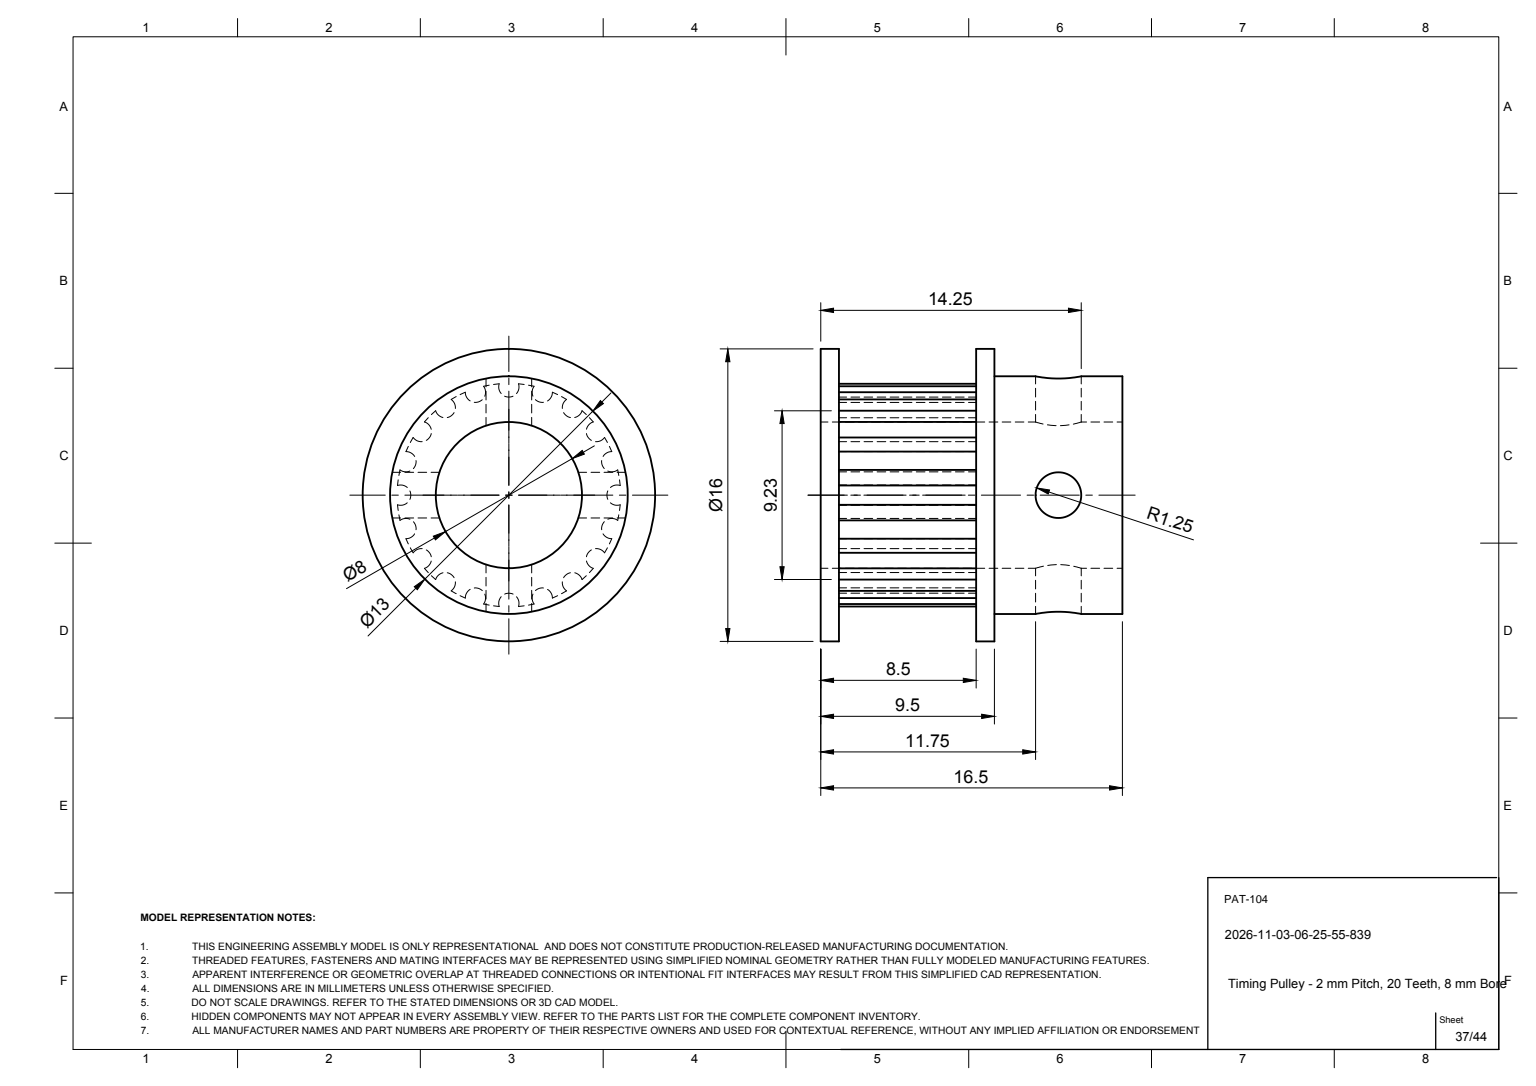
ISO-10303-21;
HEADER;
/* Generated by software containing ST-Developer
 * from STEP Tools, Inc. (www.steptools.com) 
 */

FILE_DESCRIPTION(
/* description */ ('Timing belt drive module 2 mm Pitch Timing 20T-40T'),

/* implementation_level */ '2;1');

FILE_NAME(
/* name */ 'Timing Pulley - 2 mm Pitch, 20 Teeth, 8 mm Bore.step',
/* time_stamp */ '2026-10-28T03:25:12-07:00',
/* author */ (''),
/* organization */ (''),
/* preprocessor_version */ 'ST-DEVELOPER v20.2',
/* originating_system */ 'Autodesk Translation Framework v15.17.0.0',
/* authorisation */ '');

FILE_SCHEMA (('AUTOMOTIVE_DESIGN { 1 0 10303 214 3 1 1 }'));
ENDSEC;

DATA;
#10=MECHANICAL_DESIGN_GEOMETRIC_PRESENTATION_REPRESENTATION('',(#573),#17830);
#341=B_SPLINE_CURVE_WITH_KNOTS('',3,(#16064,#16065,#16066,#16067,#16068,
#16069,#16070,#16071,#16072,#16073),.UNSPECIFIED.,.F.,.F.,(4,2,2,2,4),(0.566550474129931,
0.613761886174531,0.66097329821913,0.708186965196186,0.755400632173242),
 .UNSPECIFIED.);
#342=B_SPLINE_CURVE_WITH_KNOTS('',3,(#16075,#16076,#16077,#16078,#16079,
#16080,#16081,#16082,#16083,#16084,#16085,#16086,#16087,#16088,#16089,#16090,
#16091,#16092),.UNSPECIFIED.,.F.,.F.,(4,2,2,2,2,2,2,2,4),(0.18885015804331,
0.23606157008791,0.283272982132509,0.330486649109565,0.377700316086621,
0.424913983063677,0.472127650040732,0.519339062085332,0.566550474129931),
 .UNSPECIFIED.);
#343=B_SPLINE_CURVE_WITH_KNOTS('',3,(#16093,#16094,#16095,#16096,#16097,
#16098,#16099,#16100,#16101,#16102),.UNSPECIFIED.,.F.,.F.,(4,2,2,2,4),(0.755400632173242,
0.802614299150298,0.849827966127353,0.897039378171953,0.944250790216552),
 .UNSPECIFIED.);
#344=B_SPLINE_CURVE_WITH_KNOTS('',3,(#16106,#16107,#16108,#16109,#16110,
#16111,#16112,#16113,#16114,#16115),.UNSPECIFIED.,.F.,.F.,(4,2,2,2,4),(0.189723673274825,
0.237146208024627,0.28456874277443,0.33200804466204,0.37944734654965),
 .UNSPECIFIED.);
#345=B_SPLINE_CURVE_WITH_KNOTS('',3,(#16117,#16118,#16119,#16120,#16121,
#16122,#16123,#16124,#16125,#16126),.UNSPECIFIED.,.F.,.F.,(4,2,2,2,4),(0.,
0.0474393018876097,0.0948786037752193,0.142301138525022,0.189723673274825),
 .UNSPECIFIED.);
#346=B_SPLINE_CURVE_WITH_KNOTS('',3,(#16128,#16129,#16130,#16131,#16132,
#16133,#16134,#16135,#16136,#16137),.UNSPECIFIED.,.F.,.F.,(4,2,2,2,4),(0.569171019824474,
0.616593554574277,0.66401608932408,0.711455391211689,0.758894693099299),
 .UNSPECIFIED.);
#347=B_SPLINE_CURVE_WITH_KNOTS('',3,(#16138,#16139,#16140,#16141,#16142,
#16143,#16144,#16145,#16146,#16147),.UNSPECIFIED.,.F.,.F.,(4,2,2,2,4),(0.37944734654965,
0.426886648437259,0.474325950324869,0.521748485074671,0.569171019824474),
 .UNSPECIFIED.);
#348=B_SPLINE_CURVE_WITH_KNOTS('',3,(#16151,#16152,#16153,#16154,#16155,
#16156,#16157,#16158,#16159,#16160,#16161,#16162,#16163,#16164,#16165,#16166,
#16167,#16168),.UNSPECIFIED.,.F.,.F.,(4,2,2,2,2,2,2,2,4),(0.,0.0474393018876097,
0.0948786037752194,0.142301138525022,0.189723673274825,0.237146208024628,
0.28456874277443,0.33200804466204,0.37944734654965),.UNSPECIFIED.);
#349=B_SPLINE_CURVE_WITH_KNOTS('',3,(#16169,#16170,#16171,#16172,#16173,
#16174,#16175,#16176,#16177,#16178,#16179,#16180,#16181,#16182,#16183,#16184,
#16185,#16186),.UNSPECIFIED.,.F.,.F.,(4,2,2,2,2,2,2,2,4),(0.37944734654965,
0.426886648437259,0.474325950324869,0.521748485074672,0.569171019824474,
0.616593554574277,0.66401608932408,0.711455391211689,0.758894693099299),
 .UNSPECIFIED.);
#350=B_SPLINE_CURVE_WITH_KNOTS('',3,(#16190,#16191,#16192,#16193,#16194,
#16195,#16196,#16197,#16198,#16199),.UNSPECIFIED.,.F.,.F.,(4,2,2,2,4),(0.566550474129931,
0.613761886174531,0.66097329821913,0.708186965196186,0.755400632173242),
 .UNSPECIFIED.);
#351=B_SPLINE_CURVE_WITH_KNOTS('',3,(#16201,#16202,#16203,#16204,#16205,
#16206,#16207,#16208,#16209,#16210,#16211,#16212,#16213,#16214,#16215,#16216,
#16217,#16218),.UNSPECIFIED.,.F.,.F.,(4,2,2,2,2,2,2,2,4),(0.188850158043311,
0.23606157008791,0.283272982132509,0.330486649109565,0.377700316086621,
0.424913983063677,0.472127650040733,0.519339062085332,0.566550474129931),
 .UNSPECIFIED.);
#352=B_SPLINE_CURVE_WITH_KNOTS('',3,(#16219,#16220,#16221,#16222,#16223,
#16224,#16225,#16226,#16227,#16228),.UNSPECIFIED.,.F.,.F.,(4,2,2,2,4),(0.755400632173242,
0.802614299150298,0.849827966127354,0.897039378171953,0.944250790216552),
 .UNSPECIFIED.);
#353=B_SPLINE_CURVE_WITH_KNOTS('',3,(#16238,#16239,#16240,#16241,#16242,
#16243,#16244,#16245,#16246,#16247,#16248,#16249,#16250,#16251,#16252,#16253,
#16254,#16255),.UNSPECIFIED.,.F.,.F.,(4,2,2,2,2,2,2,2,4),(0.18885015804331,
0.23606157008791,0.283272982132509,0.330486649109565,0.377700316086621,
0.424913983063677,0.472127650040732,0.519339062085332,0.566550474129931),
 .UNSPECIFIED.);
#354=B_SPLINE_CURVE_WITH_KNOTS('',3,(#16257,#16258,#16259,#16260,#16261,
#16262,#16263,#16264,#16265,#16266),.UNSPECIFIED.,.F.,.F.,(4,2,2,2,4),(0.566550474129931,
0.613761886174531,0.66097329821913,0.708186965196186,0.755400632173242),
 .UNSPECIFIED.);
#355=B_SPLINE_CURVE_WITH_KNOTS('',3,(#16267,#16268,#16269,#16270,#16271,
#16272,#16273,#16274,#16275,#16276),.UNSPECIFIED.,.F.,.F.,(4,2,2,2,4),(0.755400632173242,
0.802614299150298,0.849827966127353,0.897039378171953,0.944250790216552),
 .UNSPECIFIED.);
#356=B_SPLINE_CURVE_WITH_KNOTS('',3,(#16279,#16280,#16281,#16282,#16283,
#16284,#16285,#16286,#16287,#16288,#16289,#16290,#16291,#16292,#16293,#16294,
#16295,#16296),.UNSPECIFIED.,.F.,.F.,(4,2,2,2,2,2,2,2,4),(0.188850158043311,
0.23606157008791,0.283272982132509,0.330486649109565,0.377700316086621,
0.424913983063677,0.472127650040733,0.519339062085332,0.566550474129932),
 .UNSPECIFIED.);
#357=B_SPLINE_CURVE_WITH_KNOTS('',3,(#16298,#16299,#16300,#16301,#16302,
#16303,#16304,#16305,#16306,#16307),.UNSPECIFIED.,.F.,.F.,(4,2,2,2,4),(0.566550474129932,
0.613761886174531,0.66097329821913,0.708186965196186,0.755400632173242),
 .UNSPECIFIED.);
#358=B_SPLINE_CURVE_WITH_KNOTS('',3,(#16308,#16309,#16310,#16311,#16312,
#16313,#16314,#16315,#16316,#16317),.UNSPECIFIED.,.F.,.F.,(4,2,2,2,4),(0.755400632173242,
0.802614299150298,0.849827966127354,0.897039378171953,0.944250790216552),
 .UNSPECIFIED.);
#359=B_SPLINE_CURVE_WITH_KNOTS('',3,(#16322,#16323,#16324,#16325,#16326,
#16327,#16328,#16329,#16330,#16331,#16332,#16333,#16334,#16335,#16336,#16337,
#16338,#16339),.UNSPECIFIED.,.F.,.F.,(4,2,2,2,2,2,2,2,4),(0.,0.0474393018876097,
0.0948786037752193,0.142301138525022,0.189723673274825,0.237146208024627,
0.28456874277443,0.33200804466204,0.37944734654965),.UNSPECIFIED.);
#360=B_SPLINE_CURVE_WITH_KNOTS('',3,(#16340,#16341,#16342,#16343,#16344,
#16345,#16346,#16347,#16348,#16349,#16350,#16351,#16352,#16353,#16354,#16355,
#16356,#16357),.UNSPECIFIED.,.F.,.F.,(4,2,2,2,2,2,2,2,4),(0.37944734654965,
0.426886648437259,0.474325950324869,0.521748485074672,0.569171019824474,
0.616593554574277,0.66401608932408,0.711455391211689,0.758894693099299),
 .UNSPECIFIED.);
#361=B_SPLINE_CURVE_WITH_KNOTS('',3,(#16361,#16362,#16363,#16364,#16365,
#16366,#16367,#16368,#16369,#16370,#16371,#16372,#16373,#16374,#16375,#16376,
#16377,#16378),.UNSPECIFIED.,.F.,.F.,(4,2,2,2,2,2,2,2,4),(0.,0.0474393018876097,
0.0948786037752194,0.142301138525022,0.189723673274825,0.237146208024627,
0.28456874277443,0.33200804466204,0.37944734654965),.UNSPECIFIED.);
#362=B_SPLINE_CURVE_WITH_KNOTS('',3,(#16379,#16380,#16381,#16382,#16383,
#16384,#16385,#16386,#16387,#16388,#16389,#16390,#16391,#16392,#16393,#16394,
#16395,#16396),.UNSPECIFIED.,.F.,.F.,(4,2,2,2,2,2,2,2,4),(0.37944734654965,
0.426886648437259,0.474325950324869,0.521748485074672,0.569171019824474,
0.616593554574277,0.66401608932408,0.711455391211689,0.758894693099299),
 .UNSPECIFIED.);
#472=SHAPE_REPRESENTATION_RELATIONSHIP('SRR','None',#18045,#515);
#515=ADVANCED_BREP_SHAPE_REPRESENTATION('',(#629),#17820);
#573=STYLED_ITEM('',(#18331),#629);
#629=MANIFOLD_SOLID_BREP('Body1',#9032);
#741=FACE_BOUND('',#1921,.T.);
#742=FACE_BOUND('',#1922,.T.);
#743=FACE_BOUND('',#1923,.T.);
#744=FACE_BOUND('',#1927,.T.);
#745=FACE_BOUND('',#1928,.T.);
#746=FACE_BOUND('',#1929,.T.);
#747=FACE_BOUND('',#1931,.T.);
#748=FACE_BOUND('',#1933,.T.);
#749=FACE_BOUND('',#1936,.T.);
#750=FACE_BOUND('',#1938,.T.);
#751=FACE_BOUND('',#1941,.T.);
#926=PLANE('',#10269);
#927=PLANE('',#10270);
#928=PLANE('',#10314);
#929=PLANE('',#10315);
#930=PLANE('',#10359);
#1293=FACE_OUTER_BOUND('',#1918,.T.);
#1294=FACE_OUTER_BOUND('',#1919,.T.);
#1295=FACE_OUTER_BOUND('',#1920,.T.);
#1296=FACE_OUTER_BOUND('',#1924,.T.);
#1297=FACE_OUTER_BOUND('',#1925,.T.);
#1298=FACE_OUTER_BOUND('',#1926,.T.);
#1299=FACE_OUTER_BOUND('',#1930,.T.);
#1300=FACE_OUTER_BOUND('',#1932,.T.);
#1301=FACE_OUTER_BOUND('',#1934,.T.);
#1302=FACE_OUTER_BOUND('',#1935,.T.);
#1303=FACE_OUTER_BOUND('',#1937,.T.);
#1304=FACE_OUTER_BOUND('',#1939,.T.);
#1305=FACE_OUTER_BOUND('',#1940,.T.);
#1306=FACE_OUTER_BOUND('',#1942,.T.);
#1307=FACE_OUTER_BOUND('',#1943,.T.);
#1308=FACE_OUTER_BOUND('',#1944,.T.);
#1309=FACE_OUTER_BOUND('',#1945,.T.);
#1310=FACE_OUTER_BOUND('',#1946,.T.);
#1311=FACE_OUTER_BOUND('',#1947,.T.);
#1312=FACE_OUTER_BOUND('',#1948,.T.);
#1313=FACE_OUTER_BOUND('',#1949,.T.);
#1314=FACE_OUTER_BOUND('',#1950,.T.);
#1315=FACE_OUTER_BOUND('',#1951,.T.);
#1316=FACE_OUTER_BOUND('',#1952,.T.);
#1317=FACE_OUTER_BOUND('',#1953,.T.);
#1318=FACE_OUTER_BOUND('',#1954,.T.);
#1319=FACE_OUTER_BOUND('',#1955,.T.);
#1320=FACE_OUTER_BOUND('',#1956,.T.);
#1321=FACE_OUTER_BOUND('',#1957,.T.);
#1322=FACE_OUTER_BOUND('',#1958,.T.);
#1323=FACE_OUTER_BOUND('',#1959,.T.);
#1324=FACE_OUTER_BOUND('',#1960,.T.);
#1325=FACE_OUTER_BOUND('',#1961,.T.);
#1326=FACE_OUTER_BOUND('',#1962,.T.);
#1327=FACE_OUTER_BOUND('',#1963,.T.);
#1328=FACE_OUTER_BOUND('',#1964,.T.);
#1329=FACE_OUTER_BOUND('',#1965,.T.);
#1330=FACE_OUTER_BOUND('',#1966,.T.);
#1331=FACE_OUTER_BOUND('',#1967,.T.);
#1332=FACE_OUTER_BOUND('',#1968,.T.);
#1333=FACE_OUTER_BOUND('',#1969,.T.);
#1334=FACE_OUTER_BOUND('',#1970,.T.);
#1335=FACE_OUTER_BOUND('',#1971,.T.);
#1336=FACE_OUTER_BOUND('',#1972,.T.);
#1337=FACE_OUTER_BOUND('',#1973,.T.);
#1338=FACE_OUTER_BOUND('',#1974,.T.);
#1339=FACE_OUTER_BOUND('',#1975,.T.);
#1340=FACE_OUTER_BOUND('',#1976,.T.);
#1341=FACE_OUTER_BOUND('',#1977,.T.);
#1342=FACE_OUTER_BOUND('',#1978,.T.);
#1343=FACE_OUTER_BOUND('',#1979,.T.);
#1344=FACE_OUTER_BOUND('',#1980,.T.);
#1345=FACE_OUTER_BOUND('',#1981,.T.);
#1918=EDGE_LOOP('',(#7165,#7166,#7167,#7168,#7169,#7170,#7171,#7172,#7173));
#1919=EDGE_LOOP('',(#7174,#7175,#7176,#7177,#7178,#7179,#7180));
#1920=EDGE_LOOP('',(#7181,#7182,#7183,#7184,#7185,#7186,#7187,#7188,#7189));
#1921=EDGE_LOOP('',(#7190,#7191,#7192));
#1922=EDGE_LOOP('',(#7193,#7194,#7195));
#1923=EDGE_LOOP('',(#7196,#7197,#7198));
#1924=EDGE_LOOP('',(#7199,#7200,#7201,#7202,#7203,#7204,#7205));
#1925=EDGE_LOOP('',(#7206,#7207,#7208,#7209,#7210,#7211,#7212));
#1926=EDGE_LOOP('',(#7213,#7214,#7215,#7216,#7217,#7218,#7219,#7220,#7221,
#7222));
#1927=EDGE_LOOP('',(#7223,#7224));
#1928=EDGE_LOOP('',(#7225,#7226));
#1929=EDGE_LOOP('',(#7227,#7228));
#1930=EDGE_LOOP('',(#7229));
#1931=EDGE_LOOP('',(#7230));
#1932=EDGE_LOOP('',(#7231));
#1933=EDGE_LOOP('',(#7232,#7233,#7234,#7235,#7236,#7237,#7238,#7239,#7240,
#7241,#7242,#7243,#7244,#7245,#7246,#7247,#7248,#7249,#7250,#7251,#7252,
#7253,#7254,#7255,#7256,#7257,#7258,#7259,#7260,#7261,#7262,#7263,#7264,
#7265,#7266,#7267,#7268,#7269,#7270,#7271));
#1934=EDGE_LOOP('',(#7272,#7273,#7274,#7275));
#1935=EDGE_LOOP('',(#7276));
#1936=EDGE_LOOP('',(#7277));
#1937=EDGE_LOOP('',(#7278));
#1938=EDGE_LOOP('',(#7279,#7280,#7281,#7282,#7283,#7284,#7285,#7286,#7287,
#7288,#7289,#7290,#7291,#7292,#7293,#7294,#7295,#7296,#7297,#7298,#7299,
#7300,#7301,#7302,#7303,#7304,#7305,#7306,#7307,#7308,#7309,#7310,#7311,
#7312,#7313,#7314,#7315,#7316,#7317,#7318));
#1939=EDGE_LOOP('',(#7319,#7320,#7321,#7322));
#1940=EDGE_LOOP('',(#7323));
#1941=EDGE_LOOP('',(#7324));
#1942=EDGE_LOOP('',(#7325,#7326,#7327,#7328));
#1943=EDGE_LOOP('',(#7329,#7330,#7331,#7332));
#1944=EDGE_LOOP('',(#7333,#7334,#7335,#7336));
#1945=EDGE_LOOP('',(#7337,#7338,#7339,#7340));
#1946=EDGE_LOOP('',(#7341,#7342,#7343,#7344));
#1947=EDGE_LOOP('',(#7345,#7346,#7347,#7348));
#1948=EDGE_LOOP('',(#7349,#7350,#7351,#7352));
#1949=EDGE_LOOP('',(#7353,#7354,#7355,#7356));
#1950=EDGE_LOOP('',(#7357,#7358,#7359,#7360));
#1951=EDGE_LOOP('',(#7361,#7362,#7363,#7364));
#1952=EDGE_LOOP('',(#7365,#7366,#7367,#7368));
#1953=EDGE_LOOP('',(#7369,#7370,#7371,#7372));
#1954=EDGE_LOOP('',(#7373,#7374,#7375,#7376));
#1955=EDGE_LOOP('',(#7377,#7378,#7379,#7380));
#1956=EDGE_LOOP('',(#7381,#7382,#7383,#7384));
#1957=EDGE_LOOP('',(#7385,#7386,#7387,#7388));
#1958=EDGE_LOOP('',(#7389,#7390,#7391,#7392));
#1959=EDGE_LOOP('',(#7393,#7394,#7395,#7396));
#1960=EDGE_LOOP('',(#7397,#7398,#7399,#7400));
#1961=EDGE_LOOP('',(#7401,#7402,#7403,#7404));
#1962=EDGE_LOOP('',(#7405,#7406,#7407,#7408));
#1963=EDGE_LOOP('',(#7409,#7410,#7411,#7412));
#1964=EDGE_LOOP('',(#7413,#7414,#7415,#7416));
#1965=EDGE_LOOP('',(#7417,#7418,#7419,#7420));
#1966=EDGE_LOOP('',(#7421,#7422,#7423,#7424));
#1967=EDGE_LOOP('',(#7425,#7426,#7427,#7428));
#1968=EDGE_LOOP('',(#7429,#7430,#7431,#7432));
#1969=EDGE_LOOP('',(#7433,#7434,#7435,#7436));
#1970=EDGE_LOOP('',(#7437,#7438,#7439,#7440));
#1971=EDGE_LOOP('',(#7441,#7442,#7443,#7444));
#1972=EDGE_LOOP('',(#7445,#7446,#7447,#7448));
#1973=EDGE_LOOP('',(#7449,#7450,#7451,#7452));
#1974=EDGE_LOOP('',(#7453,#7454,#7455,#7456));
#1975=EDGE_LOOP('',(#7457,#7458,#7459,#7460));
#1976=EDGE_LOOP('',(#7461,#7462,#7463,#7464));
#1977=EDGE_LOOP('',(#7465,#7466,#7467,#7468));
#1978=EDGE_LOOP('',(#7469,#7470,#7471,#7472));
#1979=EDGE_LOOP('',(#7473,#7474,#7475,#7476));
#1980=EDGE_LOOP('',(#7477,#7478,#7479,#7480));
#1981=EDGE_LOOP('',(#7481,#7482,#7483,#7484));
#2502=CIRCLE('',#10262,0.65);
#2503=CIRCLE('',#10263,0.65);
#2504=CIRCLE('',#10267,0.4);
#2505=CIRCLE('',#10268,0.4);
#2506=CIRCLE('',#10271,0.8);
#2507=CIRCLE('',#10272,0.0555);
#2508=CIRCLE('',#10273,0.611219772367581);
#2509=CIRCLE('',#10274,0.0555);
#2510=CIRCLE('',#10275,0.611219772367581);
#2511=CIRCLE('',#10276,0.0555);
#2512=CIRCLE('',#10277,0.611219772367581);
#2513=CIRCLE('',#10278,0.0555);
#2514=CIRCLE('',#10279,0.611219772367581);
#2515=CIRCLE('',#10280,0.0555);
#2516=CIRCLE('',#10281,0.611219772367581);
#2517=CIRCLE('',#10282,0.0555);
#2518=CIRCLE('',#10283,0.611219772367581);
#2519=CIRCLE('',#10284,0.0555);
#2520=CIRCLE('',#10285,0.611219772367581);
#2521=CIRCLE('',#10286,0.0555);
#2522=CIRCLE('',#10287,0.611219772367581);
#2523=CIRCLE('',#10288,0.0555);
#2524=CIRCLE('',#10289,0.611219772367581);
#2525=CIRCLE('',#10290,0.0555);
#2526=CIRCLE('',#10291,0.611219772367581);
#2527=CIRCLE('',#10292,0.0555);
#2528=CIRCLE('',#10293,0.611219772367581);
#2529=CIRCLE('',#10294,0.0555);
#2530=CIRCLE('',#10295,0.611219772367581);
#2531=CIRCLE('',#10296,0.0555);
#2532=CIRCLE('',#10297,0.611219772367581);
#2533=CIRCLE('',#10298,0.0555);
#2534=CIRCLE('',#10299,0.611219772367581);
#2535=CIRCLE('',#10300,0.0555);
#2536=CIRCLE('',#10301,0.611219772367581);
#2537=CIRCLE('',#10302,0.0555);
#2538=CIRCLE('',#10303,0.611219772367581);
#2539=CIRCLE('',#10304,0.0555);
#2540=CIRCLE('',#10305,0.611219772367581);
#2541=CIRCLE('',#10306,0.0555);
#2542=CIRCLE('',#10307,0.611219772367581);
#2543=CIRCLE('',#10308,0.0555);
#2544=CIRCLE('',#10309,0.611219772367581);
#2545=CIRCLE('',#10310,0.0555);
#2546=CIRCLE('',#10311,0.611219772367581);
#2547=CIRCLE('',#10313,0.8);
#2548=CIRCLE('',#10316,0.8);
#2549=CIRCLE('',#10317,0.0555);
#2550=CIRCLE('',#10318,0.611219772367581);
#2551=CIRCLE('',#10319,0.0555);
#2552=CIRCLE('',#10320,0.611219772367581);
#2553=CIRCLE('',#10321,0.0555);
#2554=CIRCLE('',#10322,0.611219772367581);
#2555=CIRCLE('',#10323,0.0555);
#2556=CIRCLE('',#10324,0.611219772367581);
#2557=CIRCLE('',#10325,0.0555);
#2558=CIRCLE('',#10326,0.611219772367581);
#2559=CIRCLE('',#10327,0.0555);
#2560=CIRCLE('',#10328,0.611219772367581);
#2561=CIRCLE('',#10329,0.0555);
#2562=CIRCLE('',#10330,0.611219772367581);
#2563=CIRCLE('',#10331,0.0555);
#2564=CIRCLE('',#10332,0.611219772367581);
#2565=CIRCLE('',#10333,0.0555);
#2566=CIRCLE('',#10334,0.611219772367581);
#2567=CIRCLE('',#10335,0.0555);
#2568=CIRCLE('',#10336,0.611219772367581);
#2569=CIRCLE('',#10337,0.0555);
#2570=CIRCLE('',#10338,0.611219772367581);
#2571=CIRCLE('',#10339,0.0555);
#2572=CIRCLE('',#10340,0.611219772367581);
#2573=CIRCLE('',#10341,0.0555);
#2574=CIRCLE('',#10342,0.611219772367581);
#2575=CIRCLE('',#10343,0.0555);
#2576=CIRCLE('',#10344,0.611219772367581);
#2577=CIRCLE('',#10345,0.0555);
#2578=CIRCLE('',#10346,0.611219772367581);
#2579=CIRCLE('',#10347,0.0555);
#2580=CIRCLE('',#10348,0.611219772367581);
#2581=CIRCLE('',#10349,0.0555);
#2582=CIRCLE('',#10350,0.611219772367581);
#2583=CIRCLE('',#10351,0.0555);
#2584=CIRCLE('',#10352,0.611219772367581);
#2585=CIRCLE('',#10353,0.0555);
#2586=CIRCLE('',#10354,0.611219772367581);
#2587=CIRCLE('',#10355,0.0555);
#2588=CIRCLE('',#10356,0.611219772367581);
#2589=CIRCLE('',#10358,0.8);
#3092=LINE('',#16104,#3570);
#3093=LINE('',#16188,#3571);
#3094=LINE('',#16232,#3572);
#3095=LINE('',#16234,#3573);
#3096=LINE('',#16320,#3574);
#3097=LINE('',#16397,#3575);
#3098=LINE('',#16401,#3576);
#3099=LINE('',#16403,#3577);
#3100=LINE('',#16492,#3578);
#3101=LINE('',#16580,#3579);
#3102=LINE('',#16583,#3580);
#3103=LINE('',#16584,#3581);
#3104=LINE('',#16586,#3582);
#3105=LINE('',#16588,#3583);
#3106=LINE('',#16590,#3584);
#3107=LINE('',#16592,#3585);
#3108=LINE('',#16594,#3586);
#3109=LINE('',#16596,#3587);
#3110=LINE('',#16598,#3588);
#3111=LINE('',#16600,#3589);
#3112=LINE('',#16602,#3590);
#3113=LINE('',#16604,#3591);
#3114=LINE('',#16606,#3592);
#3115=LINE('',#16608,#3593);
#3116=LINE('',#16610,#3594);
#3117=LINE('',#16612,#3595);
#3118=LINE('',#16614,#3596);
#3119=LINE('',#16616,#3597);
#3120=LINE('',#16618,#3598);
#3121=LINE('',#16620,#3599);
#3122=LINE('',#16622,#3600);
#3123=LINE('',#16624,#3601);
#3124=LINE('',#16626,#3602);
#3125=LINE('',#16628,#3603);
#3126=LINE('',#16630,#3604);
#3127=LINE('',#16632,#3605);
#3128=LINE('',#16634,#3606);
#3129=LINE('',#16636,#3607);
#3130=LINE('',#16638,#3608);
#3131=LINE('',#16640,#3609);
#3132=LINE('',#16642,#3610);
#3133=LINE('',#16644,#3611);
#3134=LINE('',#16646,#3612);
#3135=LINE('',#16648,#3613);
#3136=LINE('',#16650,#3614);
#3137=LINE('',#16652,#3615);
#3138=LINE('',#16654,#3616);
#3139=LINE('',#16656,#3617);
#3140=LINE('',#16658,#3618);
#3141=LINE('',#16660,#3619);
#3570=VECTOR('',#12599,0.125);
#3571=VECTOR('',#12602,0.125);
#3572=VECTOR('',#12607,0.65);
#3573=VECTOR('',#12608,0.65);
#3574=VECTOR('',#12613,0.125);
#3575=VECTOR('',#12616,0.125);
#3576=VECTOR('',#12621,0.4);
#3577=VECTOR('',#12622,0.4);
#3578=VECTOR('',#12715,0.8);
#3579=VECTOR('',#12806,0.8);
#3580=VECTOR('',#12811,1.);
#3581=VECTOR('',#12812,1.);
#3582=VECTOR('',#12815,1.);
#3583=VECTOR('',#12818,1.);
#3584=VECTOR('',#12821,1.);
#3585=VECTOR('',#12824,1.);
#3586=VECTOR('',#12827,1.);
#3587=VECTOR('',#12830,1.);
#3588=VECTOR('',#12833,1.);
#3589=VECTOR('',#12836,1.);
#3590=VECTOR('',#12839,1.);
#3591=VECTOR('',#12842,1.);
#3592=VECTOR('',#12845,1.);
#3593=VECTOR('',#12848,1.);
#3594=VECTOR('',#12851,1.);
#3595=VECTOR('',#12854,1.);
#3596=VECTOR('',#12857,1.);
#3597=VECTOR('',#12860,1.);
#3598=VECTOR('',#12863,1.);
#3599=VECTOR('',#12866,1.);
#3600=VECTOR('',#12869,1.);
#3601=VECTOR('',#12872,1.);
#3602=VECTOR('',#12875,1.);
#3603=VECTOR('',#12878,1.);
#3604=VECTOR('',#12881,1.);
#3605=VECTOR('',#12884,1.);
#3606=VECTOR('',#12887,1.);
#3607=VECTOR('',#12890,1.);
#3608=VECTOR('',#12893,1.);
#3609=VECTOR('',#12896,1.);
#3610=VECTOR('',#12899,1.);
#3611=VECTOR('',#12902,1.);
#3612=VECTOR('',#12905,1.);
#3613=VECTOR('',#12908,1.);
#3614=VECTOR('',#12911,1.);
#3615=VECTOR('',#12914,1.);
#3616=VECTOR('',#12917,1.);
#3617=VECTOR('',#12920,1.);
#3618=VECTOR('',#12923,1.);
#3619=VECTOR('',#12926,1.);
#4225=VERTEX_POINT('',#16062);
#4226=VERTEX_POINT('',#16063);
#4227=VERTEX_POINT('',#16074);
#4228=VERTEX_POINT('',#16103);
#4229=VERTEX_POINT('',#16105);
#4230=VERTEX_POINT('',#16116);
#4231=VERTEX_POINT('',#16127);
#4232=VERTEX_POINT('',#16149);
#4233=VERTEX_POINT('',#16150);
#4234=VERTEX_POINT('',#16187);
#4235=VERTEX_POINT('',#16189);
#4236=VERTEX_POINT('',#16200);
#4237=VERTEX_POINT('',#16230);
#4238=VERTEX_POINT('',#16233);
#4239=VERTEX_POINT('',#16236);
#4240=VERTEX_POINT('',#16237);
#4241=VERTEX_POINT('',#16256);
#4242=VERTEX_POINT('',#16277);
#4243=VERTEX_POINT('',#16278);
#4244=VERTEX_POINT('',#16297);
#4245=VERTEX_POINT('',#16319);
#4246=VERTEX_POINT('',#16321);
#4247=VERTEX_POINT('',#16359);
#4248=VERTEX_POINT('',#16360);
#4249=VERTEX_POINT('',#16399);
#4250=VERTEX_POINT('',#16402);
#4251=VERTEX_POINT('',#16407);
#4252=VERTEX_POINT('',#16409);
#4253=VERTEX_POINT('',#16410);
#4254=VERTEX_POINT('',#16412);
#4255=VERTEX_POINT('',#16414);
#4256=VERTEX_POINT('',#16416);
#4257=VERTEX_POINT('',#16418);
#4258=VERTEX_POINT('',#16420);
#4259=VERTEX_POINT('',#16422);
#4260=VERTEX_POINT('',#16424);
#4261=VERTEX_POINT('',#16426);
#4262=VERTEX_POINT('',#16428);
#4263=VERTEX_POINT('',#16430);
#4264=VERTEX_POINT('',#16432);
#4265=VERTEX_POINT('',#16434);
#4266=VERTEX_POINT('',#16436);
#4267=VERTEX_POINT('',#16438);
#4268=VERTEX_POINT('',#16440);
#4269=VERTEX_POINT('',#16442);
#4270=VERTEX_POINT('',#16444);
#4271=VERTEX_POINT('',#16446);
#4272=VERTEX_POINT('',#16448);
#4273=VERTEX_POINT('',#16450);
#4274=VERTEX_POINT('',#16452);
#4275=VERTEX_POINT('',#16454);
#4276=VERTEX_POINT('',#16456);
#4277=VERTEX_POINT('',#16458);
#4278=VERTEX_POINT('',#16460);
#4279=VERTEX_POINT('',#16462);
#4280=VERTEX_POINT('',#16464);
#4281=VERTEX_POINT('',#16466);
#4282=VERTEX_POINT('',#16468);
#4283=VERTEX_POINT('',#16470);
#4284=VERTEX_POINT('',#16472);
#4285=VERTEX_POINT('',#16474);
#4286=VERTEX_POINT('',#16476);
#4287=VERTEX_POINT('',#16478);
#4288=VERTEX_POINT('',#16480);
#4289=VERTEX_POINT('',#16482);
#4290=VERTEX_POINT('',#16484);
#4291=VERTEX_POINT('',#16486);
#4292=VERTEX_POINT('',#16490);
#4293=VERTEX_POINT('',#16495);
#4294=VERTEX_POINT('',#16497);
#4295=VERTEX_POINT('',#16498);
#4296=VERTEX_POINT('',#16500);
#4297=VERTEX_POINT('',#16502);
#4298=VERTEX_POINT('',#16504);
#4299=VERTEX_POINT('',#16506);
#4300=VERTEX_POINT('',#16508);
#4301=VERTEX_POINT('',#16510);
#4302=VERTEX_POINT('',#16512);
#4303=VERTEX_POINT('',#16514);
#4304=VERTEX_POINT('',#16516);
#4305=VERTEX_POINT('',#16518);
#4306=VERTEX_POINT('',#16520);
#4307=VERTEX_POINT('',#16522);
#4308=VERTEX_POINT('',#16524);
#4309=VERTEX_POINT('',#16526);
#4310=VERTEX_POINT('',#16528);
#4311=VERTEX_POINT('',#16530);
#4312=VERTEX_POINT('',#16532);
#4313=VERTEX_POINT('',#16534);
#4314=VERTEX_POINT('',#16536);
#4315=VERTEX_POINT('',#16538);
#4316=VERTEX_POINT('',#16540);
#4317=VERTEX_POINT('',#16542);
#4318=VERTEX_POINT('',#16544);
#4319=VERTEX_POINT('',#16546);
#4320=VERTEX_POINT('',#16548);
#4321=VERTEX_POINT('',#16550);
#4322=VERTEX_POINT('',#16552);
#4323=VERTEX_POINT('',#16554);
#4324=VERTEX_POINT('',#16556);
#4325=VERTEX_POINT('',#16558);
#4326=VERTEX_POINT('',#16560);
#4327=VERTEX_POINT('',#16562);
#4328=VERTEX_POINT('',#16564);
#4329=VERTEX_POINT('',#16566);
#4330=VERTEX_POINT('',#16568);
#4331=VERTEX_POINT('',#16570);
#4332=VERTEX_POINT('',#16572);
#4333=VERTEX_POINT('',#16574);
#4334=VERTEX_POINT('',#16578);
#5265=EDGE_CURVE('',#4225,#4226,#341,.T.);
#5266=EDGE_CURVE('',#4227,#4225,#342,.T.);
#5267=EDGE_CURVE('',#4226,#4227,#343,.T.);
#5268=EDGE_CURVE('',#4226,#4228,#3092,.T.);
#5269=EDGE_CURVE('',#4229,#4228,#344,.T.);
#5270=EDGE_CURVE('',#4230,#4229,#345,.T.);
#5271=EDGE_CURVE('',#4231,#4230,#346,.T.);
#5272=EDGE_CURVE('',#4228,#4231,#347,.T.);
#5273=EDGE_CURVE('',#4232,#4233,#348,.T.);
#5274=EDGE_CURVE('',#4233,#4232,#349,.T.);
#5275=EDGE_CURVE('',#4233,#4234,#3093,.T.);
#5276=EDGE_CURVE('',#4235,#4234,#350,.T.);
#5277=EDGE_CURVE('',#4236,#4235,#351,.T.);
#5278=EDGE_CURVE('',#4234,#4236,#352,.T.);
#5279=EDGE_CURVE('',#4237,#4237,#2502,.T.);
#5280=EDGE_CURVE('',#4237,#4227,#3094,.T.);
#5281=EDGE_CURVE('',#4225,#4238,#3095,.T.);
#5282=EDGE_CURVE('',#4238,#4238,#2503,.T.);
#5283=EDGE_CURVE('',#4239,#4240,#353,.T.);
#5284=EDGE_CURVE('',#4240,#4241,#354,.T.);
#5285=EDGE_CURVE('',#4241,#4239,#355,.T.);
#5286=EDGE_CURVE('',#4242,#4243,#356,.T.);
#5287=EDGE_CURVE('',#4243,#4244,#357,.T.);
#5288=EDGE_CURVE('',#4244,#4242,#358,.T.);
#5289=EDGE_CURVE('',#4241,#4245,#3096,.T.);
#5290=EDGE_CURVE('',#4246,#4245,#359,.T.);
#5291=EDGE_CURVE('',#4245,#4246,#360,.T.);
#5292=EDGE_CURVE('',#4247,#4248,#361,.T.);
#5293=EDGE_CURVE('',#4248,#4247,#362,.T.);
#5294=EDGE_CURVE('',#4248,#4244,#3097,.T.);
#5295=EDGE_CURVE('',#4249,#4249,#2504,.T.);
#5296=EDGE_CURVE('',#4249,#4229,#3098,.T.);
#5297=EDGE_CURVE('',#4231,#4250,#3099,.T.);
#5298=EDGE_CURVE('',#4250,#4250,#2505,.T.);
#5299=EDGE_CURVE('',#4251,#4251,#2506,.T.);
#5300=EDGE_CURVE('',#4252,#4253,#2507,.T.);
#5301=EDGE_CURVE('',#4254,#4253,#2508,.T.);
#5302=EDGE_CURVE('',#4254,#4255,#2509,.T.);
#5303=EDGE_CURVE('',#4256,#4255,#2510,.T.);
#5304=EDGE_CURVE('',#4256,#4257,#2511,.T.);
#5305=EDGE_CURVE('',#4258,#4257,#2512,.T.);
#5306=EDGE_CURVE('',#4258,#4259,#2513,.T.);
#5307=EDGE_CURVE('',#4260,#4259,#2514,.T.);
#5308=EDGE_CURVE('',#4260,#4261,#2515,.T.);
#5309=EDGE_CURVE('',#4262,#4261,#2516,.T.);
#5310=EDGE_CURVE('',#4262,#4263,#2517,.T.);
#5311=EDGE_CURVE('',#4264,#4263,#2518,.T.);
#5312=EDGE_CURVE('',#4264,#4265,#2519,.T.);
#5313=EDGE_CURVE('',#4266,#4265,#2520,.T.);
#5314=EDGE_CURVE('',#4266,#4267,#2521,.T.);
#5315=EDGE_CURVE('',#4268,#4267,#2522,.T.);
#5316=EDGE_CURVE('',#4268,#4269,#2523,.T.);
#5317=EDGE_CURVE('',#4270,#4269,#2524,.T.);
#5318=EDGE_CURVE('',#4270,#4271,#2525,.T.);
#5319=EDGE_CURVE('',#4272,#4271,#2526,.T.);
#5320=EDGE_CURVE('',#4272,#4273,#2527,.T.);
#5321=EDGE_CURVE('',#4274,#4273,#2528,.T.);
#5322=EDGE_CURVE('',#4274,#4275,#2529,.T.);
#5323=EDGE_CURVE('',#4276,#4275,#2530,.T.);
#5324=EDGE_CURVE('',#4276,#4277,#2531,.T.);
#5325=EDGE_CURVE('',#4278,#4277,#2532,.T.);
#5326=EDGE_CURVE('',#4278,#4279,#2533,.T.);
#5327=EDGE_CURVE('',#4280,#4279,#2534,.T.);
#5328=EDGE_CURVE('',#4280,#4281,#2535,.T.);
#5329=EDGE_CURVE('',#4282,#4281,#2536,.T.);
#5330=EDGE_CURVE('',#4282,#4283,#2537,.T.);
#5331=EDGE_CURVE('',#4284,#4283,#2538,.T.);
#5332=EDGE_CURVE('',#4284,#4285,#2539,.T.);
#5333=EDGE_CURVE('',#4286,#4285,#2540,.T.);
#5334=EDGE_CURVE('',#4286,#4287,#2541,.T.);
#5335=EDGE_CURVE('',#4288,#4287,#2542,.T.);
#5336=EDGE_CURVE('',#4288,#4289,#2543,.T.);
#5337=EDGE_CURVE('',#4290,#4289,#2544,.T.);
#5338=EDGE_CURVE('',#4290,#4291,#2545,.T.);
#5339=EDGE_CURVE('',#4252,#4291,#2546,.T.);
#5340=EDGE_CURVE('',#4292,#4292,#2547,.T.);
#5341=EDGE_CURVE('',#4292,#4251,#3100,.T.);
#5342=EDGE_CURVE('',#4293,#4293,#2548,.T.);
#5343=EDGE_CURVE('',#4294,#4295,#2549,.T.);
#5344=EDGE_CURVE('',#4295,#4296,#2550,.T.);
#5345=EDGE_CURVE('',#4296,#4297,#2551,.T.);
#5346=EDGE_CURVE('',#4297,#4298,#2552,.T.);
#5347=EDGE_CURVE('',#4298,#4299,#2553,.T.);
#5348=EDGE_CURVE('',#4299,#4300,#2554,.T.);
#5349=EDGE_CURVE('',#4300,#4301,#2555,.T.);
#5350=EDGE_CURVE('',#4301,#4302,#2556,.T.);
#5351=EDGE_CURVE('',#4302,#4303,#2557,.T.);
#5352=EDGE_CURVE('',#4303,#4304,#2558,.T.);
#5353=EDGE_CURVE('',#4304,#4305,#2559,.T.);
#5354=EDGE_CURVE('',#4305,#4306,#2560,.T.);
#5355=EDGE_CURVE('',#4306,#4307,#2561,.T.);
#5356=EDGE_CURVE('',#4307,#4308,#2562,.T.);
#5357=EDGE_CURVE('',#4308,#4309,#2563,.T.);
#5358=EDGE_CURVE('',#4309,#4310,#2564,.T.);
#5359=EDGE_CURVE('',#4310,#4311,#2565,.T.);
#5360=EDGE_CURVE('',#4311,#4312,#2566,.T.);
#5361=EDGE_CURVE('',#4312,#4313,#2567,.T.);
#5362=EDGE_CURVE('',#4313,#4314,#2568,.T.);
#5363=EDGE_CURVE('',#4314,#4315,#2569,.T.);
#5364=EDGE_CURVE('',#4315,#4316,#2570,.T.);
#5365=EDGE_CURVE('',#4316,#4317,#2571,.T.);
#5366=EDGE_CURVE('',#4317,#4318,#2572,.T.);
#5367=EDGE_CURVE('',#4318,#4319,#2573,.T.);
#5368=EDGE_CURVE('',#4319,#4320,#2574,.T.);
#5369=EDGE_CURVE('',#4320,#4321,#2575,.T.);
#5370=EDGE_CURVE('',#4321,#4322,#2576,.T.);
#5371=EDGE_CURVE('',#4322,#4323,#2577,.T.);
#5372=EDGE_CURVE('',#4323,#4324,#2578,.T.);
#5373=EDGE_CURVE('',#4324,#4325,#2579,.T.);
#5374=EDGE_CURVE('',#4325,#4326,#2580,.T.);
#5375=EDGE_CURVE('',#4326,#4327,#2581,.T.);
#5376=EDGE_CURVE('',#4327,#4328,#2582,.T.);
#5377=EDGE_CURVE('',#4328,#4329,#2583,.T.);
#5378=EDGE_CURVE('',#4329,#4330,#2584,.T.);
#5379=EDGE_CURVE('',#4330,#4331,#2585,.T.);
#5380=EDGE_CURVE('',#4331,#4332,#2586,.T.);
#5381=EDGE_CURVE('',#4332,#4333,#2587,.T.);
#5382=EDGE_CURVE('',#4333,#4294,#2588,.T.);
#5383=EDGE_CURVE('',#4334,#4334,#2589,.T.);
#5384=EDGE_CURVE('',#4334,#4293,#3101,.T.);
#5385=EDGE_CURVE('',#4295,#4252,#3102,.T.);
#5386=EDGE_CURVE('',#4253,#4294,#3103,.T.);
#5387=EDGE_CURVE('',#4333,#4254,#3104,.T.);
#5388=EDGE_CURVE('',#4255,#4332,#3105,.T.);
#5389=EDGE_CURVE('',#4331,#4256,#3106,.T.);
#5390=EDGE_CURVE('',#4257,#4330,#3107,.T.);
#5391=EDGE_CURVE('',#4329,#4258,#3108,.T.);
#5392=EDGE_CURVE('',#4259,#4328,#3109,.T.);
#5393=EDGE_CURVE('',#4327,#4260,#3110,.T.);
#5394=EDGE_CURVE('',#4261,#4326,#3111,.T.);
#5395=EDGE_CURVE('',#4325,#4262,#3112,.T.);
#5396=EDGE_CURVE('',#4263,#4324,#3113,.T.);
#5397=EDGE_CURVE('',#4323,#4264,#3114,.T.);
#5398=EDGE_CURVE('',#4265,#4322,#3115,.T.);
#5399=EDGE_CURVE('',#4321,#4266,#3116,.T.);
#5400=EDGE_CURVE('',#4267,#4320,#3117,.T.);
#5401=EDGE_CURVE('',#4319,#4268,#3118,.T.);
#5402=EDGE_CURVE('',#4269,#4318,#3119,.T.);
#5403=EDGE_CURVE('',#4317,#4270,#3120,.T.);
#5404=EDGE_CURVE('',#4271,#4316,#3121,.T.);
#5405=EDGE_CURVE('',#4315,#4272,#3122,.T.);
#5406=EDGE_CURVE('',#4273,#4314,#3123,.T.);
#5407=EDGE_CURVE('',#4313,#4274,#3124,.T.);
#5408=EDGE_CURVE('',#4275,#4312,#3125,.T.);
#5409=EDGE_CURVE('',#4311,#4276,#3126,.T.);
#5410=EDGE_CURVE('',#4277,#4310,#3127,.T.);
#5411=EDGE_CURVE('',#4309,#4278,#3128,.T.);
#5412=EDGE_CURVE('',#4279,#4308,#3129,.T.);
#5413=EDGE_CURVE('',#4307,#4280,#3130,.T.);
#5414=EDGE_CURVE('',#4281,#4306,#3131,.T.);
#5415=EDGE_CURVE('',#4305,#4282,#3132,.T.);
#5416=EDGE_CURVE('',#4283,#4304,#3133,.T.);
#5417=EDGE_CURVE('',#4303,#4284,#3134,.T.);
#5418=EDGE_CURVE('',#4285,#4302,#3135,.T.);
#5419=EDGE_CURVE('',#4301,#4286,#3136,.T.);
#5420=EDGE_CURVE('',#4287,#4300,#3137,.T.);
#5421=EDGE_CURVE('',#4299,#4288,#3138,.T.);
#5422=EDGE_CURVE('',#4289,#4298,#3139,.T.);
#5423=EDGE_CURVE('',#4291,#4296,#3140,.T.);
#5424=EDGE_CURVE('',#4297,#4290,#3141,.T.);
#7165=ORIENTED_EDGE('',*,*,#5265,.F.);
#7166=ORIENTED_EDGE('',*,*,#5266,.F.);
#7167=ORIENTED_EDGE('',*,*,#5267,.F.);
#7168=ORIENTED_EDGE('',*,*,#5268,.T.);
#7169=ORIENTED_EDGE('',*,*,#5269,.F.);
#7170=ORIENTED_EDGE('',*,*,#5270,.F.);
#7171=ORIENTED_EDGE('',*,*,#5271,.F.);
#7172=ORIENTED_EDGE('',*,*,#5272,.F.);
#7173=ORIENTED_EDGE('',*,*,#5268,.F.);
#7174=ORIENTED_EDGE('',*,*,#5273,.F.);
#7175=ORIENTED_EDGE('',*,*,#5274,.F.);
#7176=ORIENTED_EDGE('',*,*,#5275,.T.);
#7177=ORIENTED_EDGE('',*,*,#5276,.F.);
#7178=ORIENTED_EDGE('',*,*,#5277,.F.);
#7179=ORIENTED_EDGE('',*,*,#5278,.F.);
#7180=ORIENTED_EDGE('',*,*,#5275,.F.);
#7181=ORIENTED_EDGE('',*,*,#5279,.F.);
#7182=ORIENTED_EDGE('',*,*,#5280,.T.);
#7183=ORIENTED_EDGE('',*,*,#5266,.T.);
#7184=ORIENTED_EDGE('',*,*,#5281,.T.);
#7185=ORIENTED_EDGE('',*,*,#5282,.F.);
#7186=ORIENTED_EDGE('',*,*,#5281,.F.);
#7187=ORIENTED_EDGE('',*,*,#5265,.T.);
#7188=ORIENTED_EDGE('',*,*,#5267,.T.);
#7189=ORIENTED_EDGE('',*,*,#5280,.F.);
#7190=ORIENTED_EDGE('',*,*,#5277,.T.);
#7191=ORIENTED_EDGE('',*,*,#5276,.T.);
#7192=ORIENTED_EDGE('',*,*,#5278,.T.);
#7193=ORIENTED_EDGE('',*,*,#5283,.T.);
#7194=ORIENTED_EDGE('',*,*,#5284,.T.);
#7195=ORIENTED_EDGE('',*,*,#5285,.T.);
#7196=ORIENTED_EDGE('',*,*,#5286,.T.);
#7197=ORIENTED_EDGE('',*,*,#5287,.T.);
#7198=ORIENTED_EDGE('',*,*,#5288,.T.);
#7199=ORIENTED_EDGE('',*,*,#5284,.F.);
#7200=ORIENTED_EDGE('',*,*,#5283,.F.);
#7201=ORIENTED_EDGE('',*,*,#5285,.F.);
#7202=ORIENTED_EDGE('',*,*,#5289,.T.);
#7203=ORIENTED_EDGE('',*,*,#5290,.F.);
#7204=ORIENTED_EDGE('',*,*,#5291,.F.);
#7205=ORIENTED_EDGE('',*,*,#5289,.F.);
#7206=ORIENTED_EDGE('',*,*,#5292,.F.);
#7207=ORIENTED_EDGE('',*,*,#5293,.F.);
#7208=ORIENTED_EDGE('',*,*,#5294,.T.);
#7209=ORIENTED_EDGE('',*,*,#5287,.F.);
#7210=ORIENTED_EDGE('',*,*,#5286,.F.);
#7211=ORIENTED_EDGE('',*,*,#5288,.F.);
#7212=ORIENTED_EDGE('',*,*,#5294,.F.);
#7213=ORIENTED_EDGE('',*,*,#5295,.F.);
#7214=ORIENTED_EDGE('',*,*,#5296,.T.);
#7215=ORIENTED_EDGE('',*,*,#5269,.T.);
#7216=ORIENTED_EDGE('',*,*,#5272,.T.);
#7217=ORIENTED_EDGE('',*,*,#5297,.T.);
#7218=ORIENTED_EDGE('',*,*,#5298,.F.);
#7219=ORIENTED_EDGE('',*,*,#5297,.F.);
#7220=ORIENTED_EDGE('',*,*,#5271,.T.);
#7221=ORIENTED_EDGE('',*,*,#5270,.T.);
#7222=ORIENTED_EDGE('',*,*,#5296,.F.);
#7223=ORIENTED_EDGE('',*,*,#5273,.T.);
#7224=ORIENTED_EDGE('',*,*,#5274,.T.);
#7225=ORIENTED_EDGE('',*,*,#5292,.T.);
#7226=ORIENTED_EDGE('',*,*,#5293,.T.);
#7227=ORIENTED_EDGE('',*,*,#5290,.T.);
#7228=ORIENTED_EDGE('',*,*,#5291,.T.);
#7229=ORIENTED_EDGE('',*,*,#5279,.T.);
#7230=ORIENTED_EDGE('',*,*,#5295,.T.);
#7231=ORIENTED_EDGE('',*,*,#5299,.T.);
#7232=ORIENTED_EDGE('',*,*,#5300,.T.);
#7233=ORIENTED_EDGE('',*,*,#5301,.F.);
#7234=ORIENTED_EDGE('',*,*,#5302,.T.);
#7235=ORIENTED_EDGE('',*,*,#5303,.F.);
#7236=ORIENTED_EDGE('',*,*,#5304,.T.);
#7237=ORIENTED_EDGE('',*,*,#5305,.F.);
#7238=ORIENTED_EDGE('',*,*,#5306,.T.);
#7239=ORIENTED_EDGE('',*,*,#5307,.F.);
#7240=ORIENTED_EDGE('',*,*,#5308,.T.);
#7241=ORIENTED_EDGE('',*,*,#5309,.F.);
#7242=ORIENTED_EDGE('',*,*,#5310,.T.);
#7243=ORIENTED_EDGE('',*,*,#5311,.F.);
#7244=ORIENTED_EDGE('',*,*,#5312,.T.);
#7245=ORIENTED_EDGE('',*,*,#5313,.F.);
#7246=ORIENTED_EDGE('',*,*,#5314,.T.);
#7247=ORIENTED_EDGE('',*,*,#5315,.F.);
#7248=ORIENTED_EDGE('',*,*,#5316,.T.);
#7249=ORIENTED_EDGE('',*,*,#5317,.F.);
#7250=ORIENTED_EDGE('',*,*,#5318,.T.);
#7251=ORIENTED_EDGE('',*,*,#5319,.F.);
#7252=ORIENTED_EDGE('',*,*,#5320,.T.);
#7253=ORIENTED_EDGE('',*,*,#5321,.F.);
#7254=ORIENTED_EDGE('',*,*,#5322,.T.);
#7255=ORIENTED_EDGE('',*,*,#5323,.F.);
#7256=ORIENTED_EDGE('',*,*,#5324,.T.);
#7257=ORIENTED_EDGE('',*,*,#5325,.F.);
#7258=ORIENTED_EDGE('',*,*,#5326,.T.);
#7259=ORIENTED_EDGE('',*,*,#5327,.F.);
#7260=ORIENTED_EDGE('',*,*,#5328,.T.);
#7261=ORIENTED_EDGE('',*,*,#5329,.F.);
#7262=ORIENTED_EDGE('',*,*,#5330,.T.);
#7263=ORIENTED_EDGE('',*,*,#5331,.F.);
#7264=ORIENTED_EDGE('',*,*,#5332,.T.);
#7265=ORIENTED_EDGE('',*,*,#5333,.F.);
#7266=ORIENTED_EDGE('',*,*,#5334,.T.);
#7267=ORIENTED_EDGE('',*,*,#5335,.F.);
#7268=ORIENTED_EDGE('',*,*,#5336,.T.);
#7269=ORIENTED_EDGE('',*,*,#5337,.F.);
#7270=ORIENTED_EDGE('',*,*,#5338,.T.);
#7271=ORIENTED_EDGE('',*,*,#5339,.F.);
#7272=ORIENTED_EDGE('',*,*,#5340,.F.);
#7273=ORIENTED_EDGE('',*,*,#5341,.T.);
#7274=ORIENTED_EDGE('',*,*,#5299,.F.);
#7275=ORIENTED_EDGE('',*,*,#5341,.F.);
#7276=ORIENTED_EDGE('',*,*,#5340,.T.);
#7277=ORIENTED_EDGE('',*,*,#5282,.T.);
#7278=ORIENTED_EDGE('',*,*,#5342,.F.);
#7279=ORIENTED_EDGE('',*,*,#5343,.T.);
#7280=ORIENTED_EDGE('',*,*,#5344,.T.);
#7281=ORIENTED_EDGE('',*,*,#5345,.T.);
#7282=ORIENTED_EDGE('',*,*,#5346,.T.);
#7283=ORIENTED_EDGE('',*,*,#5347,.T.);
#7284=ORIENTED_EDGE('',*,*,#5348,.T.);
#7285=ORIENTED_EDGE('',*,*,#5349,.T.);
#7286=ORIENTED_EDGE('',*,*,#5350,.T.);
#7287=ORIENTED_EDGE('',*,*,#5351,.T.);
#7288=ORIENTED_EDGE('',*,*,#5352,.T.);
#7289=ORIENTED_EDGE('',*,*,#5353,.T.);
#7290=ORIENTED_EDGE('',*,*,#5354,.T.);
#7291=ORIENTED_EDGE('',*,*,#5355,.T.);
#7292=ORIENTED_EDGE('',*,*,#5356,.T.);
#7293=ORIENTED_EDGE('',*,*,#5357,.T.);
#7294=ORIENTED_EDGE('',*,*,#5358,.T.);
#7295=ORIENTED_EDGE('',*,*,#5359,.T.);
#7296=ORIENTED_EDGE('',*,*,#5360,.T.);
#7297=ORIENTED_EDGE('',*,*,#5361,.T.);
#7298=ORIENTED_EDGE('',*,*,#5362,.T.);
#7299=ORIENTED_EDGE('',*,*,#5363,.T.);
#7300=ORIENTED_EDGE('',*,*,#5364,.T.);
#7301=ORIENTED_EDGE('',*,*,#5365,.T.);
#7302=ORIENTED_EDGE('',*,*,#5366,.T.);
#7303=ORIENTED_EDGE('',*,*,#5367,.T.);
#7304=ORIENTED_EDGE('',*,*,#5368,.T.);
#7305=ORIENTED_EDGE('',*,*,#5369,.T.);
#7306=ORIENTED_EDGE('',*,*,#5370,.T.);
#7307=ORIENTED_EDGE('',*,*,#5371,.T.);
#7308=ORIENTED_EDGE('',*,*,#5372,.T.);
#7309=ORIENTED_EDGE('',*,*,#5373,.T.);
#7310=ORIENTED_EDGE('',*,*,#5374,.T.);
#7311=ORIENTED_EDGE('',*,*,#5375,.T.);
#7312=ORIENTED_EDGE('',*,*,#5376,.T.);
#7313=ORIENTED_EDGE('',*,*,#5377,.T.);
#7314=ORIENTED_EDGE('',*,*,#5378,.T.);
#7315=ORIENTED_EDGE('',*,*,#5379,.T.);
#7316=ORIENTED_EDGE('',*,*,#5380,.T.);
#7317=ORIENTED_EDGE('',*,*,#5381,.T.);
#7318=ORIENTED_EDGE('',*,*,#5382,.T.);
#7319=ORIENTED_EDGE('',*,*,#5383,.F.);
#7320=ORIENTED_EDGE('',*,*,#5384,.T.);
#7321=ORIENTED_EDGE('',*,*,#5342,.T.);
#7322=ORIENTED_EDGE('',*,*,#5384,.F.);
#7323=ORIENTED_EDGE('',*,*,#5383,.T.);
#7324=ORIENTED_EDGE('',*,*,#5298,.T.);
#7325=ORIENTED_EDGE('',*,*,#5385,.F.);
#7326=ORIENTED_EDGE('',*,*,#5343,.F.);
#7327=ORIENTED_EDGE('',*,*,#5386,.F.);
#7328=ORIENTED_EDGE('',*,*,#5300,.F.);
#7329=ORIENTED_EDGE('',*,*,#5386,.T.);
#7330=ORIENTED_EDGE('',*,*,#5382,.F.);
#7331=ORIENTED_EDGE('',*,*,#5387,.T.);
#7332=ORIENTED_EDGE('',*,*,#5301,.T.);
#7333=ORIENTED_EDGE('',*,*,#5387,.F.);
#7334=ORIENTED_EDGE('',*,*,#5381,.F.);
#7335=ORIENTED_EDGE('',*,*,#5388,.F.);
#7336=ORIENTED_EDGE('',*,*,#5302,.F.);
#7337=ORIENTED_EDGE('',*,*,#5388,.T.);
#7338=ORIENTED_EDGE('',*,*,#5380,.F.);
#7339=ORIENTED_EDGE('',*,*,#5389,.T.);
#7340=ORIENTED_EDGE('',*,*,#5303,.T.);
#7341=ORIENTED_EDGE('',*,*,#5389,.F.);
#7342=ORIENTED_EDGE('',*,*,#5379,.F.);
#7343=ORIENTED_EDGE('',*,*,#5390,.F.);
#7344=ORIENTED_EDGE('',*,*,#5304,.F.);
#7345=ORIENTED_EDGE('',*,*,#5390,.T.);
#7346=ORIENTED_EDGE('',*,*,#5378,.F.);
#7347=ORIENTED_EDGE('',*,*,#5391,.T.);
#7348=ORIENTED_EDGE('',*,*,#5305,.T.);
#7349=ORIENTED_EDGE('',*,*,#5391,.F.);
#7350=ORIENTED_EDGE('',*,*,#5377,.F.);
#7351=ORIENTED_EDGE('',*,*,#5392,.F.);
#7352=ORIENTED_EDGE('',*,*,#5306,.F.);
#7353=ORIENTED_EDGE('',*,*,#5392,.T.);
#7354=ORIENTED_EDGE('',*,*,#5376,.F.);
#7355=ORIENTED_EDGE('',*,*,#5393,.T.);
#7356=ORIENTED_EDGE('',*,*,#5307,.T.);
#7357=ORIENTED_EDGE('',*,*,#5393,.F.);
#7358=ORIENTED_EDGE('',*,*,#5375,.F.);
#7359=ORIENTED_EDGE('',*,*,#5394,.F.);
#7360=ORIENTED_EDGE('',*,*,#5308,.F.);
#7361=ORIENTED_EDGE('',*,*,#5394,.T.);
#7362=ORIENTED_EDGE('',*,*,#5374,.F.);
#7363=ORIENTED_EDGE('',*,*,#5395,.T.);
#7364=ORIENTED_EDGE('',*,*,#5309,.T.);
#7365=ORIENTED_EDGE('',*,*,#5395,.F.);
#7366=ORIENTED_EDGE('',*,*,#5373,.F.);
#7367=ORIENTED_EDGE('',*,*,#5396,.F.);
#7368=ORIENTED_EDGE('',*,*,#5310,.F.);
#7369=ORIENTED_EDGE('',*,*,#5396,.T.);
#7370=ORIENTED_EDGE('',*,*,#5372,.F.);
#7371=ORIENTED_EDGE('',*,*,#5397,.T.);
#7372=ORIENTED_EDGE('',*,*,#5311,.T.);
#7373=ORIENTED_EDGE('',*,*,#5397,.F.);
#7374=ORIENTED_EDGE('',*,*,#5371,.F.);
#7375=ORIENTED_EDGE('',*,*,#5398,.F.);
#7376=ORIENTED_EDGE('',*,*,#5312,.F.);
#7377=ORIENTED_EDGE('',*,*,#5398,.T.);
#7378=ORIENTED_EDGE('',*,*,#5370,.F.);
#7379=ORIENTED_EDGE('',*,*,#5399,.T.);
#7380=ORIENTED_EDGE('',*,*,#5313,.T.);
#7381=ORIENTED_EDGE('',*,*,#5399,.F.);
#7382=ORIENTED_EDGE('',*,*,#5369,.F.);
#7383=ORIENTED_EDGE('',*,*,#5400,.F.);
#7384=ORIENTED_EDGE('',*,*,#5314,.F.);
#7385=ORIENTED_EDGE('',*,*,#5400,.T.);
#7386=ORIENTED_EDGE('',*,*,#5368,.F.);
#7387=ORIENTED_EDGE('',*,*,#5401,.T.);
#7388=ORIENTED_EDGE('',*,*,#5315,.T.);
#7389=ORIENTED_EDGE('',*,*,#5401,.F.);
#7390=ORIENTED_EDGE('',*,*,#5367,.F.);
#7391=ORIENTED_EDGE('',*,*,#5402,.F.);
#7392=ORIENTED_EDGE('',*,*,#5316,.F.);
#7393=ORIENTED_EDGE('',*,*,#5402,.T.);
#7394=ORIENTED_EDGE('',*,*,#5366,.F.);
#7395=ORIENTED_EDGE('',*,*,#5403,.T.);
#7396=ORIENTED_EDGE('',*,*,#5317,.T.);
#7397=ORIENTED_EDGE('',*,*,#5403,.F.);
#7398=ORIENTED_EDGE('',*,*,#5365,.F.);
#7399=ORIENTED_EDGE('',*,*,#5404,.F.);
#7400=ORIENTED_EDGE('',*,*,#5318,.F.);
#7401=ORIENTED_EDGE('',*,*,#5404,.T.);
#7402=ORIENTED_EDGE('',*,*,#5364,.F.);
#7403=ORIENTED_EDGE('',*,*,#5405,.T.);
#7404=ORIENTED_EDGE('',*,*,#5319,.T.);
#7405=ORIENTED_EDGE('',*,*,#5405,.F.);
#7406=ORIENTED_EDGE('',*,*,#5363,.F.);
#7407=ORIENTED_EDGE('',*,*,#5406,.F.);
#7408=ORIENTED_EDGE('',*,*,#5320,.F.);
#7409=ORIENTED_EDGE('',*,*,#5406,.T.);
#7410=ORIENTED_EDGE('',*,*,#5362,.F.);
#7411=ORIENTED_EDGE('',*,*,#5407,.T.);
#7412=ORIENTED_EDGE('',*,*,#5321,.T.);
#7413=ORIENTED_EDGE('',*,*,#5407,.F.);
#7414=ORIENTED_EDGE('',*,*,#5361,.F.);
#7415=ORIENTED_EDGE('',*,*,#5408,.F.);
#7416=ORIENTED_EDGE('',*,*,#5322,.F.);
#7417=ORIENTED_EDGE('',*,*,#5408,.T.);
#7418=ORIENTED_EDGE('',*,*,#5360,.F.);
#7419=ORIENTED_EDGE('',*,*,#5409,.T.);
#7420=ORIENTED_EDGE('',*,*,#5323,.T.);
#7421=ORIENTED_EDGE('',*,*,#5409,.F.);
#7422=ORIENTED_EDGE('',*,*,#5359,.F.);
#7423=ORIENTED_EDGE('',*,*,#5410,.F.);
#7424=ORIENTED_EDGE('',*,*,#5324,.F.);
#7425=ORIENTED_EDGE('',*,*,#5410,.T.);
#7426=ORIENTED_EDGE('',*,*,#5358,.F.);
#7427=ORIENTED_EDGE('',*,*,#5411,.T.);
#7428=ORIENTED_EDGE('',*,*,#5325,.T.);
#7429=ORIENTED_EDGE('',*,*,#5411,.F.);
#7430=ORIENTED_EDGE('',*,*,#5357,.F.);
#7431=ORIENTED_EDGE('',*,*,#5412,.F.);
#7432=ORIENTED_EDGE('',*,*,#5326,.F.);
#7433=ORIENTED_EDGE('',*,*,#5412,.T.);
#7434=ORIENTED_EDGE('',*,*,#5356,.F.);
#7435=ORIENTED_EDGE('',*,*,#5413,.T.);
#7436=ORIENTED_EDGE('',*,*,#5327,.T.);
#7437=ORIENTED_EDGE('',*,*,#5413,.F.);
#7438=ORIENTED_EDGE('',*,*,#5355,.F.);
#7439=ORIENTED_EDGE('',*,*,#5414,.F.);
#7440=ORIENTED_EDGE('',*,*,#5328,.F.);
#7441=ORIENTED_EDGE('',*,*,#5414,.T.);
#7442=ORIENTED_EDGE('',*,*,#5354,.F.);
#7443=ORIENTED_EDGE('',*,*,#5415,.T.);
#7444=ORIENTED_EDGE('',*,*,#5329,.T.);
#7445=ORIENTED_EDGE('',*,*,#5415,.F.);
#7446=ORIENTED_EDGE('',*,*,#5353,.F.);
#7447=ORIENTED_EDGE('',*,*,#5416,.F.);
#7448=ORIENTED_EDGE('',*,*,#5330,.F.);
#7449=ORIENTED_EDGE('',*,*,#5416,.T.);
#7450=ORIENTED_EDGE('',*,*,#5352,.F.);
#7451=ORIENTED_EDGE('',*,*,#5417,.T.);
#7452=ORIENTED_EDGE('',*,*,#5331,.T.);
#7453=ORIENTED_EDGE('',*,*,#5417,.F.);
#7454=ORIENTED_EDGE('',*,*,#5351,.F.);
#7455=ORIENTED_EDGE('',*,*,#5418,.F.);
#7456=ORIENTED_EDGE('',*,*,#5332,.F.);
#7457=ORIENTED_EDGE('',*,*,#5418,.T.);
#7458=ORIENTED_EDGE('',*,*,#5350,.F.);
#7459=ORIENTED_EDGE('',*,*,#5419,.T.);
#7460=ORIENTED_EDGE('',*,*,#5333,.T.);
#7461=ORIENTED_EDGE('',*,*,#5419,.F.);
#7462=ORIENTED_EDGE('',*,*,#5349,.F.);
#7463=ORIENTED_EDGE('',*,*,#5420,.F.);
#7464=ORIENTED_EDGE('',*,*,#5334,.F.);
#7465=ORIENTED_EDGE('',*,*,#5420,.T.);
#7466=ORIENTED_EDGE('',*,*,#5348,.F.);
#7467=ORIENTED_EDGE('',*,*,#5421,.T.);
#7468=ORIENTED_EDGE('',*,*,#5335,.T.);
#7469=ORIENTED_EDGE('',*,*,#5422,.F.);
#7470=ORIENTED_EDGE('',*,*,#5336,.F.);
#7471=ORIENTED_EDGE('',*,*,#5421,.F.);
#7472=ORIENTED_EDGE('',*,*,#5347,.F.);
#7473=ORIENTED_EDGE('',*,*,#5385,.T.);
#7474=ORIENTED_EDGE('',*,*,#5339,.T.);
#7475=ORIENTED_EDGE('',*,*,#5423,.T.);
#7476=ORIENTED_EDGE('',*,*,#5344,.F.);
#7477=ORIENTED_EDGE('',*,*,#5424,.F.);
#7478=ORIENTED_EDGE('',*,*,#5345,.F.);
#7479=ORIENTED_EDGE('',*,*,#5423,.F.);
#7480=ORIENTED_EDGE('',*,*,#5338,.F.);
#7481=ORIENTED_EDGE('',*,*,#5422,.T.);
#7482=ORIENTED_EDGE('',*,*,#5346,.F.);
#7483=ORIENTED_EDGE('',*,*,#5424,.T.);
#7484=ORIENTED_EDGE('',*,*,#5337,.T.);
#8310=CYLINDRICAL_SURFACE('',#10259,0.125);
#8311=CYLINDRICAL_SURFACE('',#10260,0.125);
#8312=CYLINDRICAL_SURFACE('',#10261,0.65);
#8313=CYLINDRICAL_SURFACE('',#10264,0.125);
#8314=CYLINDRICAL_SURFACE('',#10265,0.125);
#8315=CYLINDRICAL_SURFACE('',#10266,0.4);
#8316=CYLINDRICAL_SURFACE('',#10312,0.8);
#8317=CYLINDRICAL_SURFACE('',#10357,0.8);
#8318=CYLINDRICAL_SURFACE('',#10360,0.0555);
#8319=CYLINDRICAL_SURFACE('',#10361,0.611219772367581);
#8320=CYLINDRICAL_SURFACE('',#10362,0.0555);
#8321=CYLINDRICAL_SURFACE('',#10363,0.611219772367581);
#8322=CYLINDRICAL_SURFACE('',#10364,0.0555);
#8323=CYLINDRICAL_SURFACE('',#10365,0.611219772367581);
#8324=CYLINDRICAL_SURFACE('',#10366,0.0555);
#8325=CYLINDRICAL_SURFACE('',#10367,0.611219772367581);
#8326=CYLINDRICAL_SURFACE('',#10368,0.0555);
#8327=CYLINDRICAL_SURFACE('',#10369,0.611219772367581);
#8328=CYLINDRICAL_SURFACE('',#10370,0.0555);
#8329=CYLINDRICAL_SURFACE('',#10371,0.611219772367581);
#8330=CYLINDRICAL_SURFACE('',#10372,0.0555);
#8331=CYLINDRICAL_SURFACE('',#10373,0.611219772367581);
#8332=CYLINDRICAL_SURFACE('',#10374,0.0555);
#8333=CYLINDRICAL_SURFACE('',#10375,0.611219772367581);
#8334=CYLINDRICAL_SURFACE('',#10376,0.0555);
#8335=CYLINDRICAL_SURFACE('',#10377,0.611219772367581);
#8336=CYLINDRICAL_SURFACE('',#10378,0.0555);
#8337=CYLINDRICAL_SURFACE('',#10379,0.611219772367581);
#8338=CYLINDRICAL_SURFACE('',#10380,0.0555);
#8339=CYLINDRICAL_SURFACE('',#10381,0.611219772367581);
#8340=CYLINDRICAL_SURFACE('',#10382,0.0555);
#8341=CYLINDRICAL_SURFACE('',#10383,0.611219772367581);
#8342=CYLINDRICAL_SURFACE('',#10384,0.0555);
#8343=CYLINDRICAL_SURFACE('',#10385,0.611219772367581);
#8344=CYLINDRICAL_SURFACE('',#10386,0.0555);
#8345=CYLINDRICAL_SURFACE('',#10387,0.611219772367581);
#8346=CYLINDRICAL_SURFACE('',#10388,0.0555);
#8347=CYLINDRICAL_SURFACE('',#10389,0.611219772367581);
#8348=CYLINDRICAL_SURFACE('',#10390,0.0555);
#8349=CYLINDRICAL_SURFACE('',#10391,0.611219772367581);
#8350=CYLINDRICAL_SURFACE('',#10392,0.0555);
#8351=CYLINDRICAL_SURFACE('',#10393,0.611219772367581);
#8352=CYLINDRICAL_SURFACE('',#10394,0.0555);
#8353=CYLINDRICAL_SURFACE('',#10395,0.611219772367581);
#8354=CYLINDRICAL_SURFACE('',#10396,0.0555);
#8355=CYLINDRICAL_SURFACE('',#10397,0.611219772367581);
#8356=CYLINDRICAL_SURFACE('',#10398,0.0555);
#8357=CYLINDRICAL_SURFACE('',#10399,0.611219772367581);
#8791=ADVANCED_FACE('',(#1293),#8310,.F.);
#8792=ADVANCED_FACE('',(#1294),#8311,.F.);
#8793=ADVANCED_FACE('',(#1295,#741,#742,#743),#8312,.T.);
#8794=ADVANCED_FACE('',(#1296),#8313,.F.);
#8795=ADVANCED_FACE('',(#1297),#8314,.F.);
#8796=ADVANCED_FACE('',(#1298,#744,#745,#746),#8315,.F.);
#8797=ADVANCED_FACE('',(#1299,#747),#926,.F.);
#8798=ADVANCED_FACE('',(#1300,#748),#927,.T.);
#8799=ADVANCED_FACE('',(#1301),#8316,.T.);
#8800=ADVANCED_FACE('',(#1302,#749),#928,.F.);
#8801=ADVANCED_FACE('',(#1303,#750),#929,.F.);
#8802=ADVANCED_FACE('',(#1304),#8317,.T.);
#8803=ADVANCED_FACE('',(#1305,#751),#930,.T.);
#8804=ADVANCED_FACE('',(#1306),#8318,.F.);
#8805=ADVANCED_FACE('',(#1307),#8319,.T.);
#8806=ADVANCED_FACE('',(#1308),#8320,.F.);
#8807=ADVANCED_FACE('',(#1309),#8321,.T.);
#8808=ADVANCED_FACE('',(#1310),#8322,.F.);
#8809=ADVANCED_FACE('',(#1311),#8323,.T.);
#8810=ADVANCED_FACE('',(#1312),#8324,.F.);
#8811=ADVANCED_FACE('',(#1313),#8325,.T.);
#8812=ADVANCED_FACE('',(#1314),#8326,.F.);
#8813=ADVANCED_FACE('',(#1315),#8327,.T.);
#8814=ADVANCED_FACE('',(#1316),#8328,.F.);
#8815=ADVANCED_FACE('',(#1317),#8329,.T.);
#8816=ADVANCED_FACE('',(#1318),#8330,.F.);
#8817=ADVANCED_FACE('',(#1319),#8331,.T.);
#8818=ADVANCED_FACE('',(#1320),#8332,.F.);
#8819=ADVANCED_FACE('',(#1321),#8333,.T.);
#8820=ADVANCED_FACE('',(#1322),#8334,.F.);
#8821=ADVANCED_FACE('',(#1323),#8335,.T.);
#8822=ADVANCED_FACE('',(#1324),#8336,.F.);
#8823=ADVANCED_FACE('',(#1325),#8337,.T.);
#8824=ADVANCED_FACE('',(#1326),#8338,.F.);
#8825=ADVANCED_FACE('',(#1327),#8339,.T.);
#8826=ADVANCED_FACE('',(#1328),#8340,.F.);
#8827=ADVANCED_FACE('',(#1329),#8341,.T.);
#8828=ADVANCED_FACE('',(#1330),#8342,.F.);
#8829=ADVANCED_FACE('',(#1331),#8343,.T.);
#8830=ADVANCED_FACE('',(#1332),#8344,.F.);
#8831=ADVANCED_FACE('',(#1333),#8345,.T.);
#8832=ADVANCED_FACE('',(#1334),#8346,.F.);
#8833=ADVANCED_FACE('',(#1335),#8347,.T.);
#8834=ADVANCED_FACE('',(#1336),#8348,.F.);
#8835=ADVANCED_FACE('',(#1337),#8349,.T.);
#8836=ADVANCED_FACE('',(#1338),#8350,.F.);
#8837=ADVANCED_FACE('',(#1339),#8351,.T.);
#8838=ADVANCED_FACE('',(#1340),#8352,.F.);
#8839=ADVANCED_FACE('',(#1341),#8353,.T.);
#8840=ADVANCED_FACE('',(#1342),#8354,.F.);
#8841=ADVANCED_FACE('',(#1343),#8355,.T.);
#8842=ADVANCED_FACE('',(#1344),#8356,.F.);
#8843=ADVANCED_FACE('',(#1345),#8357,.T.);
#9032=CLOSED_SHELL('',(#8791,#8792,#8793,#8794,#8795,#8796,#8797,#8798,
#8799,#8800,#8801,#8802,#8803,#8804,#8805,#8806,#8807,#8808,#8809,#8810,
#8811,#8812,#8813,#8814,#8815,#8816,#8817,#8818,#8819,#8820,#8821,#8822,
#8823,#8824,#8825,#8826,#8827,#8828,#8829,#8830,#8831,#8832,#8833,#8834,
#8835,#8836,#8837,#8838,#8839,#8840,#8841,#8842,#8843));
#10258=AXIS2_PLACEMENT_3D('',#16060,#12595,#12596);
#10259=AXIS2_PLACEMENT_3D('',#16061,#12597,#12598);
#10260=AXIS2_PLACEMENT_3D('',#16148,#12600,#12601);
#10261=AXIS2_PLACEMENT_3D('',#16229,#12603,#12604);
#10262=AXIS2_PLACEMENT_3D('',#16231,#12605,#12606);
#10263=AXIS2_PLACEMENT_3D('',#16235,#12609,#12610);
#10264=AXIS2_PLACEMENT_3D('',#16318,#12611,#12612);
#10265=AXIS2_PLACEMENT_3D('',#16358,#12614,#12615);
#10266=AXIS2_PLACEMENT_3D('',#16398,#12617,#12618);
#10267=AXIS2_PLACEMENT_3D('',#16400,#12619,#12620);
#10268=AXIS2_PLACEMENT_3D('',#16404,#12623,#12624);
#10269=AXIS2_PLACEMENT_3D('',#16405,#12625,#12626);
#10270=AXIS2_PLACEMENT_3D('',#16406,#12627,#12628);
#10271=AXIS2_PLACEMENT_3D('',#16408,#12629,#12630);
#10272=AXIS2_PLACEMENT_3D('',#16411,#12631,#12632);
#10273=AXIS2_PLACEMENT_3D('',#16413,#12633,#12634);
#10274=AXIS2_PLACEMENT_3D('',#16415,#12635,#12636);
#10275=AXIS2_PLACEMENT_3D('',#16417,#12637,#12638);
#10276=AXIS2_PLACEMENT_3D('',#16419,#12639,#12640);
#10277=AXIS2_PLACEMENT_3D('',#16421,#12641,#12642);
#10278=AXIS2_PLACEMENT_3D('',#16423,#12643,#12644);
#10279=AXIS2_PLACEMENT_3D('',#16425,#12645,#12646);
#10280=AXIS2_PLACEMENT_3D('',#16427,#12647,#12648);
#10281=AXIS2_PLACEMENT_3D('',#16429,#12649,#12650);
#10282=AXIS2_PLACEMENT_3D('',#16431,#12651,#12652);
#10283=AXIS2_PLACEMENT_3D('',#16433,#12653,#12654);
#10284=AXIS2_PLACEMENT_3D('',#16435,#12655,#12656);
#10285=AXIS2_PLACEMENT_3D('',#16437,#12657,#12658);
#10286=AXIS2_PLACEMENT_3D('',#16439,#12659,#12660);
#10287=AXIS2_PLACEMENT_3D('',#16441,#12661,#12662);
#10288=AXIS2_PLACEMENT_3D('',#16443,#12663,#12664);
#10289=AXIS2_PLACEMENT_3D('',#16445,#12665,#12666);
#10290=AXIS2_PLACEMENT_3D('',#16447,#12667,#12668);
#10291=AXIS2_PLACEMENT_3D('',#16449,#12669,#12670);
#10292=AXIS2_PLACEMENT_3D('',#16451,#12671,#12672);
#10293=AXIS2_PLACEMENT_3D('',#16453,#12673,#12674);
#10294=AXIS2_PLACEMENT_3D('',#16455,#12675,#12676);
#10295=AXIS2_PLACEMENT_3D('',#16457,#12677,#12678);
#10296=AXIS2_PLACEMENT_3D('',#16459,#12679,#12680);
#10297=AXIS2_PLACEMENT_3D('',#16461,#12681,#12682);
#10298=AXIS2_PLACEMENT_3D('',#16463,#12683,#12684);
#10299=AXIS2_PLACEMENT_3D('',#16465,#12685,#12686);
#10300=AXIS2_PLACEMENT_3D('',#16467,#12687,#12688);
#10301=AXIS2_PLACEMENT_3D('',#16469,#12689,#12690);
#10302=AXIS2_PLACEMENT_3D('',#16471,#12691,#12692);
#10303=AXIS2_PLACEMENT_3D('',#16473,#12693,#12694);
#10304=AXIS2_PLACEMENT_3D('',#16475,#12695,#12696);
#10305=AXIS2_PLACEMENT_3D('',#16477,#12697,#12698);
#10306=AXIS2_PLACEMENT_3D('',#16479,#12699,#12700);
#10307=AXIS2_PLACEMENT_3D('',#16481,#12701,#12702);
#10308=AXIS2_PLACEMENT_3D('',#16483,#12703,#12704);
#10309=AXIS2_PLACEMENT_3D('',#16485,#12705,#12706);
#10310=AXIS2_PLACEMENT_3D('',#16487,#12707,#12708);
#10311=AXIS2_PLACEMENT_3D('',#16488,#12709,#12710);
#10312=AXIS2_PLACEMENT_3D('',#16489,#12711,#12712);
#10313=AXIS2_PLACEMENT_3D('',#16491,#12713,#12714);
#10314=AXIS2_PLACEMENT_3D('',#16493,#12716,#12717);
#10315=AXIS2_PLACEMENT_3D('',#16494,#12718,#12719);
#10316=AXIS2_PLACEMENT_3D('',#16496,#12720,#12721);
#10317=AXIS2_PLACEMENT_3D('',#16499,#12722,#12723);
#10318=AXIS2_PLACEMENT_3D('',#16501,#12724,#12725);
#10319=AXIS2_PLACEMENT_3D('',#16503,#12726,#12727);
#10320=AXIS2_PLACEMENT_3D('',#16505,#12728,#12729);
#10321=AXIS2_PLACEMENT_3D('',#16507,#12730,#12731);
#10322=AXIS2_PLACEMENT_3D('',#16509,#12732,#12733);
#10323=AXIS2_PLACEMENT_3D('',#16511,#12734,#12735);
#10324=AXIS2_PLACEMENT_3D('',#16513,#12736,#12737);
#10325=AXIS2_PLACEMENT_3D('',#16515,#12738,#12739);
#10326=AXIS2_PLACEMENT_3D('',#16517,#12740,#12741);
#10327=AXIS2_PLACEMENT_3D('',#16519,#12742,#12743);
#10328=AXIS2_PLACEMENT_3D('',#16521,#12744,#12745);
#10329=AXIS2_PLACEMENT_3D('',#16523,#12746,#12747);
#10330=AXIS2_PLACEMENT_3D('',#16525,#12748,#12749);
#10331=AXIS2_PLACEMENT_3D('',#16527,#12750,#12751);
#10332=AXIS2_PLACEMENT_3D('',#16529,#12752,#12753);
#10333=AXIS2_PLACEMENT_3D('',#16531,#12754,#12755);
#10334=AXIS2_PLACEMENT_3D('',#16533,#12756,#12757);
#10335=AXIS2_PLACEMENT_3D('',#16535,#12758,#12759);
#10336=AXIS2_PLACEMENT_3D('',#16537,#12760,#12761);
#10337=AXIS2_PLACEMENT_3D('',#16539,#12762,#12763);
#10338=AXIS2_PLACEMENT_3D('',#16541,#12764,#12765);
#10339=AXIS2_PLACEMENT_3D('',#16543,#12766,#12767);
#10340=AXIS2_PLACEMENT_3D('',#16545,#12768,#12769);
#10341=AXIS2_PLACEMENT_3D('',#16547,#12770,#12771);
#10342=AXIS2_PLACEMENT_3D('',#16549,#12772,#12773);
#10343=AXIS2_PLACEMENT_3D('',#16551,#12774,#12775);
#10344=AXIS2_PLACEMENT_3D('',#16553,#12776,#12777);
#10345=AXIS2_PLACEMENT_3D('',#16555,#12778,#12779);
#10346=AXIS2_PLACEMENT_3D('',#16557,#12780,#12781);
#10347=AXIS2_PLACEMENT_3D('',#16559,#12782,#12783);
#10348=AXIS2_PLACEMENT_3D('',#16561,#12784,#12785);
#10349=AXIS2_PLACEMENT_3D('',#16563,#12786,#12787);
#10350=AXIS2_PLACEMENT_3D('',#16565,#12788,#12789);
#10351=AXIS2_PLACEMENT_3D('',#16567,#12790,#12791);
#10352=AXIS2_PLACEMENT_3D('',#16569,#12792,#12793);
#10353=AXIS2_PLACEMENT_3D('',#16571,#12794,#12795);
#10354=AXIS2_PLACEMENT_3D('',#16573,#12796,#12797);
#10355=AXIS2_PLACEMENT_3D('',#16575,#12798,#12799);
#10356=AXIS2_PLACEMENT_3D('',#16576,#12800,#12801);
#10357=AXIS2_PLACEMENT_3D('',#16577,#12802,#12803);
#10358=AXIS2_PLACEMENT_3D('',#16579,#12804,#12805);
#10359=AXIS2_PLACEMENT_3D('',#16581,#12807,#12808);
#10360=AXIS2_PLACEMENT_3D('',#16582,#12809,#12810);
#10361=AXIS2_PLACEMENT_3D('',#16585,#12813,#12814);
#10362=AXIS2_PLACEMENT_3D('',#16587,#12816,#12817);
#10363=AXIS2_PLACEMENT_3D('',#16589,#12819,#12820);
#10364=AXIS2_PLACEMENT_3D('',#16591,#12822,#12823);
#10365=AXIS2_PLACEMENT_3D('',#16593,#12825,#12826);
#10366=AXIS2_PLACEMENT_3D('',#16595,#12828,#12829);
#10367=AXIS2_PLACEMENT_3D('',#16597,#12831,#12832);
#10368=AXIS2_PLACEMENT_3D('',#16599,#12834,#12835);
#10369=AXIS2_PLACEMENT_3D('',#16601,#12837,#12838);
#10370=AXIS2_PLACEMENT_3D('',#16603,#12840,#12841);
#10371=AXIS2_PLACEMENT_3D('',#16605,#12843,#12844);
#10372=AXIS2_PLACEMENT_3D('',#16607,#12846,#12847);
#10373=AXIS2_PLACEMENT_3D('',#16609,#12849,#12850);
#10374=AXIS2_PLACEMENT_3D('',#16611,#12852,#12853);
#10375=AXIS2_PLACEMENT_3D('',#16613,#12855,#12856);
#10376=AXIS2_PLACEMENT_3D('',#16615,#12858,#12859);
#10377=AXIS2_PLACEMENT_3D('',#16617,#12861,#12862);
#10378=AXIS2_PLACEMENT_3D('',#16619,#12864,#12865);
#10379=AXIS2_PLACEMENT_3D('',#16621,#12867,#12868);
#10380=AXIS2_PLACEMENT_3D('',#16623,#12870,#12871);
#10381=AXIS2_PLACEMENT_3D('',#16625,#12873,#12874);
#10382=AXIS2_PLACEMENT_3D('',#16627,#12876,#12877);
#10383=AXIS2_PLACEMENT_3D('',#16629,#12879,#12880);
#10384=AXIS2_PLACEMENT_3D('',#16631,#12882,#12883);
#10385=AXIS2_PLACEMENT_3D('',#16633,#12885,#12886);
#10386=AXIS2_PLACEMENT_3D('',#16635,#12888,#12889);
#10387=AXIS2_PLACEMENT_3D('',#16637,#12891,#12892);
#10388=AXIS2_PLACEMENT_3D('',#16639,#12894,#12895);
#10389=AXIS2_PLACEMENT_3D('',#16641,#12897,#12898);
#10390=AXIS2_PLACEMENT_3D('',#16643,#12900,#12901);
#10391=AXIS2_PLACEMENT_3D('',#16645,#12903,#12904);
#10392=AXIS2_PLACEMENT_3D('',#16647,#12906,#12907);
#10393=AXIS2_PLACEMENT_3D('',#16649,#12909,#12910);
#10394=AXIS2_PLACEMENT_3D('',#16651,#12912,#12913);
#10395=AXIS2_PLACEMENT_3D('',#16653,#12915,#12916);
#10396=AXIS2_PLACEMENT_3D('',#16655,#12918,#12919);
#10397=AXIS2_PLACEMENT_3D('',#16657,#12921,#12922);
#10398=AXIS2_PLACEMENT_3D('',#16659,#12924,#12925);
#10399=AXIS2_PLACEMENT_3D('',#16661,#12927,#12928);
#12595=DIRECTION('axis',(0.,0.,1.));
#12596=DIRECTION('refdir',(1.,0.,0.));
#12597=DIRECTION('center_axis',(1.,0.,6.12323399573677E-17));
#12598=DIRECTION('ref_axis',(6.12323399573677E-17,0.,-1.));
#12599=DIRECTION('',(1.,0.,6.12323399573677E-17));
#12600=DIRECTION('center_axis',(1.,0.,6.12323399573677E-17));
#12601=DIRECTION('ref_axis',(6.12323399573677E-17,0.,-1.));
#12602=DIRECTION('',(1.,0.,6.12323399573677E-17));
#12603=DIRECTION('center_axis',(0.,-1.,0.));
#12604=DIRECTION('ref_axis',(1.,0.,0.));
#12605=DIRECTION('center_axis',(0.,-1.,0.));
#12606=DIRECTION('ref_axis',(1.,0.,0.));
#12607=DIRECTION('',(0.,1.,0.));
#12608=DIRECTION('',(0.,1.,0.));
#12609=DIRECTION('center_axis',(0.,1.,0.));
#12610=DIRECTION('ref_axis',(1.,0.,0.));
#12611=DIRECTION('center_axis',(0.,0.,1.));
#12612=DIRECTION('ref_axis',(1.,0.,0.));
#12613=DIRECTION('',(0.,0.,1.));
#12614=DIRECTION('center_axis',(0.,0.,1.));
#12615=DIRECTION('ref_axis',(1.,0.,0.));
#12616=DIRECTION('',(0.,0.,1.));
#12617=DIRECTION('center_axis',(0.,1.,0.));
#12618=DIRECTION('ref_axis',(1.,0.,0.));
#12619=DIRECTION('center_axis',(0.,1.,0.));
#12620=DIRECTION('ref_axis',(1.,0.,0.));
#12621=DIRECTION('',(0.,1.,0.));
#12622=DIRECTION('',(0.,1.,0.));
#12623=DIRECTION('center_axis',(0.,-1.,0.));
#12624=DIRECTION('ref_axis',(1.,0.,0.));
#12625=DIRECTION('center_axis',(0.,1.,0.));
#12626=DIRECTION('ref_axis',(1.,0.,0.));
#12627=DIRECTION('center_axis',(0.,1.,0.));
#12628=DIRECTION('ref_axis',(1.,0.,0.));
#12629=DIRECTION('center_axis',(0.,1.,0.));
#12630=DIRECTION('ref_axis',(1.,0.,0.));
#12631=DIRECTION('center_axis',(0.,1.,0.));
#12632=DIRECTION('ref_axis',(0.951056516295154,0.,0.309016994374948));
#12633=DIRECTION('center_axis',(0.,1.,0.));
#12634=DIRECTION('ref_axis',(1.,0.,0.));
#12635=DIRECTION('center_axis',(0.,1.,0.));
#12636=DIRECTION('ref_axis',(0.809016994374947,0.,0.587785252292473));
#12637=DIRECTION('center_axis',(0.,1.,0.));
#12638=DIRECTION('ref_axis',(1.,0.,0.));
#12639=DIRECTION('center_axis',(0.,1.,0.));
#12640=DIRECTION('ref_axis',(0.587785252292473,0.,0.809016994374948));
#12641=DIRECTION('center_axis',(0.,1.,0.));
#12642=DIRECTION('ref_axis',(1.,0.,0.));
#12643=DIRECTION('center_axis',(0.,1.,0.));
#12644=DIRECTION('ref_axis',(0.309016994374947,0.,0.951056516295154));
#12645=DIRECTION('center_axis',(0.,1.,0.));
#12646=DIRECTION('ref_axis',(1.,0.,0.));
#12647=DIRECTION('center_axis',(0.,1.,0.));
#12648=DIRECTION('ref_axis',(-1.83697019872103E-16,0.,1.));
#12649=DIRECTION('center_axis',(0.,1.,0.));
#12650=DIRECTION('ref_axis',(1.,0.,0.));
#12651=DIRECTION('center_axis',(0.,1.,0.));
#12652=DIRECTION('ref_axis',(-0.309016994374948,0.,0.951056516295154));
#12653=DIRECTION('center_axis',(0.,1.,0.));
#12654=DIRECTION('ref_axis',(1.,0.,0.));
#12655=DIRECTION('center_axis',(0.,1.,0.));
#12656=DIRECTION('ref_axis',(-0.587785252292473,0.,0.809016994374947));
#12657=DIRECTION('center_axis',(0.,1.,0.));
#12658=DIRECTION('ref_axis',(1.,0.,0.));
#12659=DIRECTION('center_axis',(0.,1.,0.));
#12660=DIRECTION('ref_axis',(-0.809016994374947,0.,0.587785252292473));
#12661=DIRECTION('center_axis',(0.,1.,0.));
#12662=DIRECTION('ref_axis',(1.,0.,0.));
#12663=DIRECTION('center_axis',(0.,1.,0.));
#12664=DIRECTION('ref_axis',(-0.951056516295154,0.,0.309016994374947));
#12665=DIRECTION('center_axis',(0.,1.,0.));
#12666=DIRECTION('ref_axis',(1.,0.,0.));
#12667=DIRECTION('center_axis',(0.,1.,0.));
#12668=DIRECTION('ref_axis',(-1.,0.,-1.22464679914735E-16));
#12669=DIRECTION('center_axis',(0.,1.,0.));
#12670=DIRECTION('ref_axis',(1.,0.,0.));
#12671=DIRECTION('center_axis',(0.,1.,0.));
#12672=DIRECTION('ref_axis',(-0.951056516295154,0.,-0.309016994374948));
#12673=DIRECTION('center_axis',(0.,1.,0.));
#12674=DIRECTION('ref_axis',(1.,0.,0.));
#12675=DIRECTION('center_axis',(0.,1.,0.));
#12676=DIRECTION('ref_axis',(-0.809016994374947,0.,-0.587785252292473));
#12677=DIRECTION('center_axis',(0.,1.,0.));
#12678=DIRECTION('ref_axis',(1.,0.,0.));
#12679=DIRECTION('center_axis',(0.,1.,0.));
#12680=DIRECTION('ref_axis',(-0.587785252292473,0.,-0.809016994374948));
#12681=DIRECTION('center_axis',(0.,1.,0.));
#12682=DIRECTION('ref_axis',(1.,0.,0.));
#12683=DIRECTION('center_axis',(0.,1.,0.));
#12684=DIRECTION('ref_axis',(-0.309016994374947,0.,-0.951056516295154));
#12685=DIRECTION('center_axis',(0.,1.,0.));
#12686=DIRECTION('ref_axis',(1.,0.,0.));
#12687=DIRECTION('center_axis',(0.,1.,0.));
#12688=DIRECTION('ref_axis',(6.12323399573677E-17,0.,-1.));
#12689=DIRECTION('center_axis',(0.,1.,0.));
#12690=DIRECTION('ref_axis',(1.,0.,0.));
#12691=DIRECTION('center_axis',(0.,1.,0.));
#12692=DIRECTION('ref_axis',(0.309016994374947,0.,-0.951056516295154));
#12693=DIRECTION('center_axis',(0.,1.,0.));
#12694=DIRECTION('ref_axis',(1.,0.,0.));
#12695=DIRECTION('center_axis',(0.,1.,0.));
#12696=DIRECTION('ref_axis',(0.587785252292473,0.,-0.809016994374947));
#12697=DIRECTION('center_axis',(0.,1.,0.));
#12698=DIRECTION('ref_axis',(1.,0.,0.));
#12699=DIRECTION('center_axis',(0.,1.,0.));
#12700=DIRECTION('ref_axis',(0.809016994374947,0.,-0.587785252292473));
#12701=DIRECTION('center_axis',(0.,1.,0.));
#12702=DIRECTION('ref_axis',(1.,0.,0.));
#12703=DIRECTION('center_axis',(0.,1.,0.));
#12704=DIRECTION('ref_axis',(0.951056516295154,0.,-0.309016994374947));
#12705=DIRECTION('center_axis',(0.,1.,0.));
#12706=DIRECTION('ref_axis',(1.,0.,0.));
#12707=DIRECTION('center_axis',(0.,1.,0.));
#12708=DIRECTION('ref_axis',(1.,0.,0.));
#12709=DIRECTION('center_axis',(0.,1.,0.));
#12710=DIRECTION('ref_axis',(1.,0.,0.));
#12711=DIRECTION('center_axis',(0.,-1.,0.));
#12712=DIRECTION('ref_axis',(1.,0.,0.));
#12713=DIRECTION('center_axis',(0.,-1.,0.));
#12714=DIRECTION('ref_axis',(1.,0.,0.));
#12715=DIRECTION('',(0.,1.,0.));
#12716=DIRECTION('center_axis',(0.,1.,0.));
#12717=DIRECTION('ref_axis',(1.,0.,0.));
#12718=DIRECTION('center_axis',(0.,1.,0.));
#12719=DIRECTION('ref_axis',(1.,0.,0.));
#12720=DIRECTION('center_axis',(0.,1.,0.));
#12721=DIRECTION('ref_axis',(1.,0.,0.));
#12722=DIRECTION('center_axis',(0.,-1.,0.));
#12723=DIRECTION('ref_axis',(0.951056516295154,0.,0.309016994374948));
#12724=DIRECTION('center_axis',(0.,1.,0.));
#12725=DIRECTION('ref_axis',(1.,0.,0.));
#12726=DIRECTION('center_axis',(0.,-1.,0.));
#12727=DIRECTION('ref_axis',(1.,0.,0.));
#12728=DIRECTION('center_axis',(0.,1.,0.));
#12729=DIRECTION('ref_axis',(1.,0.,0.));
#12730=DIRECTION('center_axis',(0.,-1.,0.));
#12731=DIRECTION('ref_axis',(0.951056516295154,0.,-0.309016994374947));
#12732=DIRECTION('center_axis',(0.,1.,0.));
#12733=DIRECTION('ref_axis',(1.,0.,0.));
#12734=DIRECTION('center_axis',(0.,-1.,0.));
#12735=DIRECTION('ref_axis',(0.809016994374947,0.,-0.587785252292473));
#12736=DIRECTION('center_axis',(0.,1.,0.));
#12737=DIRECTION('ref_axis',(1.,0.,0.));
#12738=DIRECTION('center_axis',(0.,-1.,0.));
#12739=DIRECTION('ref_axis',(0.587785252292473,0.,-0.809016994374947));
#12740=DIRECTION('center_axis',(0.,1.,0.));
#12741=DIRECTION('ref_axis',(1.,0.,0.));
#12742=DIRECTION('center_axis',(0.,-1.,0.));
#12743=DIRECTION('ref_axis',(0.309016994374947,0.,-0.951056516295154));
#12744=DIRECTION('center_axis',(0.,1.,0.));
#12745=DIRECTION('ref_axis',(1.,0.,0.));
#12746=DIRECTION('center_axis',(0.,-1.,0.));
#12747=DIRECTION('ref_axis',(6.12323399573677E-17,0.,-1.));
#12748=DIRECTION('center_axis',(0.,1.,0.));
#12749=DIRECTION('ref_axis',(1.,0.,0.));
#12750=DIRECTION('center_axis',(0.,-1.,0.));
#12751=DIRECTION('ref_axis',(-0.309016994374947,0.,-0.951056516295154));
#12752=DIRECTION('center_axis',(0.,1.,0.));
#12753=DIRECTION('ref_axis',(1.,0.,0.));
#12754=DIRECTION('center_axis',(0.,-1.,0.));
#12755=DIRECTION('ref_axis',(-0.587785252292473,0.,-0.809016994374948));
#12756=DIRECTION('center_axis',(0.,1.,0.));
#12757=DIRECTION('ref_axis',(1.,0.,0.));
#12758=DIRECTION('center_axis',(0.,-1.,0.));
#12759=DIRECTION('ref_axis',(-0.809016994374947,0.,-0.587785252292473));
#12760=DIRECTION('center_axis',(0.,1.,0.));
#12761=DIRECTION('ref_axis',(1.,0.,0.));
#12762=DIRECTION('center_axis',(0.,-1.,0.));
#12763=DIRECTION('ref_axis',(-0.951056516295154,0.,-0.309016994374948));
#12764=DIRECTION('center_axis',(0.,1.,0.));
#12765=DIRECTION('ref_axis',(1.,0.,0.));
#12766=DIRECTION('center_axis',(0.,-1.,0.));
#12767=DIRECTION('ref_axis',(-1.,0.,-1.22464679914735E-16));
#12768=DIRECTION('center_axis',(0.,1.,0.));
#12769=DIRECTION('ref_axis',(1.,0.,0.));
#12770=DIRECTION('center_axis',(0.,-1.,0.));
#12771=DIRECTION('ref_axis',(-0.951056516295154,0.,0.309016994374947));
#12772=DIRECTION('center_axis',(0.,1.,0.));
#12773=DIRECTION('ref_axis',(1.,0.,0.));
#12774=DIRECTION('center_axis',(0.,-1.,0.));
#12775=DIRECTION('ref_axis',(-0.809016994374947,0.,0.587785252292473));
#12776=DIRECTION('center_axis',(0.,1.,0.));
#12777=DIRECTION('ref_axis',(1.,0.,0.));
#12778=DIRECTION('center_axis',(0.,-1.,0.));
#12779=DIRECTION('ref_axis',(-0.587785252292473,0.,0.809016994374947));
#12780=DIRECTION('center_axis',(0.,1.,0.));
#12781=DIRECTION('ref_axis',(1.,0.,0.));
#12782=DIRECTION('center_axis',(0.,-1.,0.));
#12783=DIRECTION('ref_axis',(-0.309016994374948,0.,0.951056516295154));
#12784=DIRECTION('center_axis',(0.,1.,0.));
#12785=DIRECTION('ref_axis',(1.,0.,0.));
#12786=DIRECTION('center_axis',(0.,-1.,0.));
#12787=DIRECTION('ref_axis',(-1.83697019872103E-16,0.,1.));
#12788=DIRECTION('center_axis',(0.,1.,0.));
#12789=DIRECTION('ref_axis',(1.,0.,0.));
#12790=DIRECTION('center_axis',(0.,-1.,0.));
#12791=DIRECTION('ref_axis',(0.309016994374947,0.,0.951056516295154));
#12792=DIRECTION('center_axis',(0.,1.,0.));
#12793=DIRECTION('ref_axis',(1.,0.,0.));
#12794=DIRECTION('center_axis',(0.,-1.,0.));
#12795=DIRECTION('ref_axis',(0.587785252292473,0.,0.809016994374948));
#12796=DIRECTION('center_axis',(0.,1.,0.));
#12797=DIRECTION('ref_axis',(1.,0.,0.));
#12798=DIRECTION('center_axis',(0.,-1.,0.));
#12799=DIRECTION('ref_axis',(0.809016994374947,0.,0.587785252292473));
#12800=DIRECTION('center_axis',(0.,1.,0.));
#12801=DIRECTION('ref_axis',(1.,0.,0.));
#12802=DIRECTION('center_axis',(0.,1.,0.));
#12803=DIRECTION('ref_axis',(1.,0.,0.));
#12804=DIRECTION('center_axis',(0.,1.,0.));
#12805=DIRECTION('ref_axis',(1.,0.,0.));
#12806=DIRECTION('',(0.,-1.,0.));
#12807=DIRECTION('center_axis',(0.,1.,0.));
#12808=DIRECTION('ref_axis',(1.,0.,0.));
#12809=DIRECTION('center_axis',(0.,1.,0.));
#12810=DIRECTION('ref_axis',(-0.951056516295153,0.,-0.309016994374948));
#12811=DIRECTION('',(0.,-1.,0.));
#12812=DIRECTION('',(0.,1.,0.));
#12813=DIRECTION('center_axis',(0.,1.,0.));
#12814=DIRECTION('ref_axis',(1.,0.,0.));
#12815=DIRECTION('',(0.,-1.,0.));
#12816=DIRECTION('center_axis',(0.,1.,0.));
#12817=DIRECTION('ref_axis',(-0.809016994374947,0.,-0.587785252292473));
#12818=DIRECTION('',(0.,1.,0.));
#12819=DIRECTION('center_axis',(0.,1.,0.));
#12820=DIRECTION('ref_axis',(1.,0.,0.));
#12821=DIRECTION('',(0.,-1.,0.));
#12822=DIRECTION('center_axis',(0.,1.,0.));
#12823=DIRECTION('ref_axis',(-0.587785252292473,0.,-0.809016994374947));
#12824=DIRECTION('',(0.,1.,0.));
#12825=DIRECTION('center_axis',(0.,1.,0.));
#12826=DIRECTION('ref_axis',(1.,0.,0.));
#12827=DIRECTION('',(0.,-1.,0.));
#12828=DIRECTION('center_axis',(0.,1.,0.));
#12829=DIRECTION('ref_axis',(-0.309016994374947,0.,-0.951056516295154));
#12830=DIRECTION('',(0.,1.,0.));
#12831=DIRECTION('center_axis',(0.,1.,0.));
#12832=DIRECTION('ref_axis',(1.,0.,0.));
#12833=DIRECTION('',(0.,-1.,0.));
#12834=DIRECTION('center_axis',(0.,1.,0.));
#12835=DIRECTION('ref_axis',(-1.37927510063224E-16,0.,-1.));
#12836=DIRECTION('',(0.,1.,0.));
#12837=DIRECTION('center_axis',(0.,1.,0.));
#12838=DIRECTION('ref_axis',(1.,0.,0.));
#12839=DIRECTION('',(0.,-1.,0.));
#12840=DIRECTION('center_axis',(0.,1.,0.));
#12841=DIRECTION('ref_axis',(0.309016994374948,0.,-0.951056516295154));
#12842=DIRECTION('',(0.,1.,0.));
#12843=DIRECTION('center_axis',(0.,1.,0.));
#12844=DIRECTION('ref_axis',(1.,0.,0.));
#12845=DIRECTION('',(0.,-1.,0.));
#12846=DIRECTION('center_axis',(0.,1.,0.));
#12847=DIRECTION('ref_axis',(0.587785252292473,0.,-0.809016994374948));
#12848=DIRECTION('',(0.,1.,0.));
#12849=DIRECTION('center_axis',(0.,1.,0.));
#12850=DIRECTION('ref_axis',(1.,0.,0.));
#12851=DIRECTION('',(0.,-1.,0.));
#12852=DIRECTION('center_axis',(0.,1.,0.));
#12853=DIRECTION('ref_axis',(0.809016994374948,0.,-0.587785252292473));
#12854=DIRECTION('',(0.,1.,0.));
#12855=DIRECTION('center_axis',(0.,1.,0.));
#12856=DIRECTION('ref_axis',(1.,0.,0.));
#12857=DIRECTION('',(0.,-1.,0.));
#12858=DIRECTION('center_axis',(0.,1.,0.));
#12859=DIRECTION('ref_axis',(0.951056516295154,0.,-0.309016994374947));
#12860=DIRECTION('',(0.,1.,0.));
#12861=DIRECTION('center_axis',(0.,1.,0.));
#12862=DIRECTION('ref_axis',(1.,0.,0.));
#12863=DIRECTION('',(0.,-1.,0.));
#12864=DIRECTION('center_axis',(0.,1.,0.));
#12865=DIRECTION('ref_axis',(1.,0.,-1.99159850020592E-16));
#12866=DIRECTION('',(0.,1.,0.));
#12867=DIRECTION('center_axis',(0.,1.,0.));
#12868=DIRECTION('ref_axis',(1.,0.,0.));
#12869=DIRECTION('',(0.,-1.,0.));
#12870=DIRECTION('center_axis',(0.,1.,0.));
#12871=DIRECTION('ref_axis',(0.951056516295154,0.,0.309016994374948));
#12872=DIRECTION('',(0.,1.,0.));
#12873=DIRECTION('center_axis',(0.,1.,0.));
#12874=DIRECTION('ref_axis',(1.,0.,0.));
#12875=DIRECTION('',(0.,-1.,0.));
#12876=DIRECTION('center_axis',(0.,1.,0.));
#12877=DIRECTION('ref_axis',(0.809016994374948,0.,0.587785252292473));
#12878=DIRECTION('',(0.,1.,0.));
#12879=DIRECTION('center_axis',(0.,1.,0.));
#12880=DIRECTION('ref_axis',(1.,0.,0.));
#12881=DIRECTION('',(0.,-1.,0.));
#12882=DIRECTION('center_axis',(0.,1.,0.));
#12883=DIRECTION('ref_axis',(0.587785252292473,0.,0.809016994374948));
#12884=DIRECTION('',(0.,1.,0.));
#12885=DIRECTION('center_axis',(0.,1.,0.));
#12886=DIRECTION('ref_axis',(1.,0.,0.));
#12887=DIRECTION('',(0.,-1.,0.));
#12888=DIRECTION('center_axis',(0.,1.,0.));
#12889=DIRECTION('ref_axis',(0.309016994374947,0.,0.951056516295154));
#12890=DIRECTION('',(0.,1.,0.));
#12891=DIRECTION('center_axis',(0.,1.,0.));
#12892=DIRECTION('ref_axis',(1.,0.,0.));
#12893=DIRECTION('',(0.,-1.,0.));
#12894=DIRECTION('center_axis',(0.,1.,0.));
#12895=DIRECTION('ref_axis',(2.6039218997796E-16,0.,1.));
#12896=DIRECTION('',(0.,1.,0.));
#12897=DIRECTION('center_axis',(0.,1.,0.));
#12898=DIRECTION('ref_axis',(1.,0.,0.));
#12899=DIRECTION('',(0.,-1.,0.));
#12900=DIRECTION('center_axis',(0.,1.,0.));
#12901=DIRECTION('ref_axis',(-0.309016994374948,0.,0.951056516295153));
#12902=DIRECTION('',(0.,1.,0.));
#12903=DIRECTION('center_axis',(0.,1.,0.));
#12904=DIRECTION('ref_axis',(1.,0.,0.));
#12905=DIRECTION('',(0.,-1.,0.));
#12906=DIRECTION('center_axis',(0.,1.,0.));
#12907=DIRECTION('ref_axis',(-0.587785252292474,0.,0.809016994374947));
#12908=DIRECTION('',(0.,1.,0.));
#12909=DIRECTION('center_axis',(0.,1.,0.));
#12910=DIRECTION('ref_axis',(1.,0.,0.));
#12911=DIRECTION('',(0.,-1.,0.));
#12912=DIRECTION('center_axis',(0.,1.,0.));
#12913=DIRECTION('ref_axis',(-0.809016994374948,0.,0.587785252292473));
#12914=DIRECTION('',(0.,1.,0.));
#12915=DIRECTION('center_axis',(0.,1.,0.));
#12916=DIRECTION('ref_axis',(1.,0.,0.));
#12917=DIRECTION('',(0.,-1.,0.));
#12918=DIRECTION('center_axis',(0.,1.,0.));
#12919=DIRECTION('ref_axis',(-0.951056516295154,0.,0.309016994374948));
#12920=DIRECTION('',(0.,1.,0.));
#12921=DIRECTION('center_axis',(0.,1.,0.));
#12922=DIRECTION('ref_axis',(1.,0.,0.));
#12923=DIRECTION('',(0.,1.,0.));
#12924=DIRECTION('center_axis',(0.,1.,0.));
#12925=DIRECTION('ref_axis',(-1.,0.,-1.22464679914735E-16));
#12926=DIRECTION('',(0.,-1.,0.));
#12927=DIRECTION('center_axis',(0.,1.,0.));
#12928=DIRECTION('ref_axis',(1.,0.,0.));
#16060=CARTESIAN_POINT('',(0.,0.,0.));
#16061=CARTESIAN_POINT('Origin',(0.,-0.45,0.));
#16062=CARTESIAN_POINT('',(-0.65,-0.325,-3.9801020972289E-17));
#16063=CARTESIAN_POINT('',(-0.637867541108654,-0.45,0.125));
#16064=CARTESIAN_POINT('Ctrl Pts',(-0.65,-0.325,-6.93889390390723E-17));
#16065=CARTESIAN_POINT('Ctrl Pts',(-0.65,-0.325,0.0157371373481997));
#16066=CARTESIAN_POINT('Ctrl Pts',(-0.649370620646074,-0.328153081062251,
0.0324967135411163));
#16067=CARTESIAN_POINT('Ctrl Pts',(-0.647096224417991,-0.340922081922822,
0.0632828231545122));
#16068=CARTESIAN_POINT('Ctrl Pts',(-0.645482573914132,-0.350535859112198,
0.0773125544088347));
#16069=CARTESIAN_POINT('Ctrl Pts',(-0.642442040715078,-0.372687974598127,
0.0994646698947638));
#16070=CARTESIAN_POINT('Ctrl Pts',(-0.640815160902589,-0.386717480603274,
0.109078032552995));
#16071=CARTESIAN_POINT('Ctrl Pts',(-0.63851034608138,-0.417502809542363,
0.121846732641678));
#16072=CARTESIAN_POINT('Ctrl Pts',(-0.637867541108654,-0.434262111007648,
0.125));
#16073=CARTESIAN_POINT('Ctrl Pts',(-0.637867541108654,-0.45,0.125));
#16074=CARTESIAN_POINT('',(-0.65,-0.575,-3.9801020972289E-17));
#16075=CARTESIAN_POINT('Ctrl Pts',(-0.65,-0.575,-3.46944695195361E-18));
#16076=CARTESIAN_POINT('Ctrl Pts',(-0.65,-0.575,-0.0157371373481998));
#16077=CARTESIAN_POINT('Ctrl Pts',(-0.649370620646074,-0.571846918937749,
-0.0324967135411164));
#16078=CARTESIAN_POINT('Ctrl Pts',(-0.647096224417991,-0.559077918077178,
-0.0632828231545123));
#16079=CARTESIAN_POINT('Ctrl Pts',(-0.645482573914132,-0.549464140887802,
-0.0773125544088349));
#16080=CARTESIAN_POINT('Ctrl Pts',(-0.642442040715078,-0.527312025401873,
-0.099464669894764));
#16081=CARTESIAN_POINT('Ctrl Pts',(-0.640815160902589,-0.513282519396725,
-0.109078032552995));
#16082=CARTESIAN_POINT('Ctrl Pts',(-0.63851034608138,-0.482497190457637,
-0.121846732641678));
#16083=CARTESIAN_POINT('Ctrl Pts',(-0.637867541108654,-0.465737888992352,
-0.125));
#16084=CARTESIAN_POINT('Ctrl Pts',(-0.637867541108654,-0.434262111007648,
-0.125));
#16085=CARTESIAN_POINT('Ctrl Pts',(-0.63851034608138,-0.417502809542363,
-0.121846732641678));
#16086=CARTESIAN_POINT('Ctrl Pts',(-0.640815160902589,-0.386717480603275,
-0.109078032552995));
#16087=CARTESIAN_POINT('Ctrl Pts',(-0.642442040715078,-0.372687974598127,
-0.099464669894764));
#16088=CARTESIAN_POINT('Ctrl Pts',(-0.645482573914132,-0.350535859112198,
-0.077312554408835));
#16089=CARTESIAN_POINT('Ctrl Pts',(-0.647096224417991,-0.340922081922822,
-0.0632828231545124));
#16090=CARTESIAN_POINT('Ctrl Pts',(-0.649370620646074,-0.328153081062251,
-0.0324967135411165));
#16091=CARTESIAN_POINT('Ctrl Pts',(-0.65,-0.325,-0.0157371373481999));
#16092=CARTESIAN_POINT('Ctrl Pts',(-0.65,-0.325,-8.32667268468867E-17));
#16093=CARTESIAN_POINT('Ctrl Pts',(-0.637867541108654,-0.45,0.125));
#16094=CARTESIAN_POINT('Ctrl Pts',(-0.637867541108654,-0.465737888992352,
0.125));
#16095=CARTESIAN_POINT('Ctrl Pts',(-0.63851034608138,-0.482497190457637,
0.121846732641678));
#16096=CARTESIAN_POINT('Ctrl Pts',(-0.640815160902589,-0.513282519396725,
0.109078032552995));
#16097=CARTESIAN_POINT('Ctrl Pts',(-0.642442040715078,-0.527312025401873,
0.0994646698947639));
#16098=CARTESIAN_POINT('Ctrl Pts',(-0.645482573914132,-0.549464140887802,
0.0773125544088349));
#16099=CARTESIAN_POINT('Ctrl Pts',(-0.647096224417991,-0.559077918077178,
0.0632828231545123));
#16100=CARTESIAN_POINT('Ctrl Pts',(-0.649370620646074,-0.571846918937749,
0.0324967135411164));
#16101=CARTESIAN_POINT('Ctrl Pts',(-0.65,-0.575,0.0157371373481998));
#16102=CARTESIAN_POINT('Ctrl Pts',(-0.65,-0.575,-2.08166817117217E-17));
#16103=CARTESIAN_POINT('',(-0.379967103839267,-0.45,0.125));
#16104=CARTESIAN_POINT('',(-7.65404249467096E-18,-0.45,0.125));
#16105=CARTESIAN_POINT('',(-0.4,-0.575,5.41097774720219E-18));
#16106=CARTESIAN_POINT('Ctrl Pts',(-0.4,-0.575,-3.81639164714898E-17));
#16107=CARTESIAN_POINT('Ctrl Pts',(-0.4,-0.575,0.0158075115832675));
#16108=CARTESIAN_POINT('Ctrl Pts',(-0.398970551469948,-0.571819306519379,
0.0325978607437828));
#16109=CARTESIAN_POINT('Ctrl Pts',(-0.395252954914593,-0.559029081159106,
0.0633657881355917));
#16110=CARTESIAN_POINT('Ctrl Pts',(-0.392612801026882,-0.549425200318011,
0.0773514949786256));
#16111=CARTESIAN_POINT('Ctrl Pts',(-0.38761064154154,-0.527347592689753,
0.0994291026068839));
#16112=CARTESIAN_POINT('Ctrl Pts',(-0.384911758361269,-0.51336346023721,
0.109029967924066));
#16113=CARTESIAN_POINT('Ctrl Pts',(-0.381057715344782,-0.48260129709332,
0.121817958968287));
#16114=CARTESIAN_POINT('Ctrl Pts',(-0.379967103839267,-0.465813100629203,
0.125));
#16115=CARTESIAN_POINT('Ctrl Pts',(-0.379967103839267,-0.45,0.125));
#16116=CARTESIAN_POINT('',(-0.379967103839267,-0.45,-0.125));
#16117=CARTESIAN_POINT('Ctrl Pts',(-0.379967103839267,-0.45,-0.125));
#16118=CARTESIAN_POINT('Ctrl Pts',(-0.379967103839267,-0.465813100629203,
-0.125));
#16119=CARTESIAN_POINT('Ctrl Pts',(-0.381057715344782,-0.48260129709332,
-0.121817958968287));
#16120=CARTESIAN_POINT('Ctrl Pts',(-0.384911758361269,-0.51336346023721,
-0.109029967924066));
#16121=CARTESIAN_POINT('Ctrl Pts',(-0.38761064154154,-0.527347592689753,
-0.099429102606884));
#16122=CARTESIAN_POINT('Ctrl Pts',(-0.392612801026882,-0.549425200318011,
-0.0773514949786257));
#16123=CARTESIAN_POINT('Ctrl Pts',(-0.395252954914593,-0.559029081159106,
-0.0633657881355918));
#16124=CARTESIAN_POINT('Ctrl Pts',(-0.398970551469948,-0.571819306519379,
-0.0325978607437828));
#16125=CARTESIAN_POINT('Ctrl Pts',(-0.4,-0.575,-0.0158075115832676));
#16126=CARTESIAN_POINT('Ctrl Pts',(-0.4,-0.575,-4.16333634234434E-17));
#16127=CARTESIAN_POINT('',(-0.4,-0.325,2.96971064108775E-17));
#16128=CARTESIAN_POINT('Ctrl Pts',(-0.4,-0.325,1.04083408558608E-17));
#16129=CARTESIAN_POINT('Ctrl Pts',(-0.4,-0.325,-0.0158075115832676));
#16130=CARTESIAN_POINT('Ctrl Pts',(-0.398970551469948,-0.328180693480621,
-0.0325978607437828));
#16131=CARTESIAN_POINT('Ctrl Pts',(-0.395252954914593,-0.340970918840894,
-0.0633657881355918));
#16132=CARTESIAN_POINT('Ctrl Pts',(-0.392612801026882,-0.350574799681989,
-0.0773514949786256));
#16133=CARTESIAN_POINT('Ctrl Pts',(-0.38761064154154,-0.372652407310247,
-0.0994291026068839));
#16134=CARTESIAN_POINT('Ctrl Pts',(-0.384911758361269,-0.38663653976279,
-0.109029967924066));
#16135=CARTESIAN_POINT('Ctrl Pts',(-0.381057715344782,-0.41739870290668,
-0.121817958968287));
#16136=CARTESIAN_POINT('Ctrl Pts',(-0.379967103839267,-0.434186899370797,
-0.125));
#16137=CARTESIAN_POINT('Ctrl Pts',(-0.379967103839267,-0.45,-0.125));
#16138=CARTESIAN_POINT('Ctrl Pts',(-0.379967103839267,-0.45,0.125));
#16139=CARTESIAN_POINT('Ctrl Pts',(-0.379967103839267,-0.434186899370797,
0.125));
#16140=CARTESIAN_POINT('Ctrl Pts',(-0.381057715344782,-0.41739870290668,
0.121817958968287));
#16141=CARTESIAN_POINT('Ctrl Pts',(-0.384911758361269,-0.38663653976279,
0.109029967924066));
#16142=CARTESIAN_POINT('Ctrl Pts',(-0.38761064154154,-0.372652407310247,
0.0994291026068839));
#16143=CARTESIAN_POINT('Ctrl Pts',(-0.392612801026882,-0.350574799681989,
0.0773514949786257));
#16144=CARTESIAN_POINT('Ctrl Pts',(-0.395252954914593,-0.340970918840894,
0.0633657881355918));
#16145=CARTESIAN_POINT('Ctrl Pts',(-0.398970551469948,-0.328180693480621,
0.0325978607437829));
#16146=CARTESIAN_POINT('Ctrl Pts',(-0.4,-0.325,0.0158075115832676));
#16147=CARTESIAN_POINT('Ctrl Pts',(-0.4,-0.325,1.38777878078145E-17));
#16148=CARTESIAN_POINT('Origin',(0.,-0.45,0.));
#16149=CARTESIAN_POINT('',(0.379967103839267,-0.45,-0.125));
#16150=CARTESIAN_POINT('',(0.379967103839267,-0.45,0.125));
#16151=CARTESIAN_POINT('Ctrl Pts',(0.379967103839267,-0.45,-0.125));
#16152=CARTESIAN_POINT('Ctrl Pts',(0.379967103839267,-0.434186899370797,
-0.125));
#16153=CARTESIAN_POINT('Ctrl Pts',(0.381057715344782,-0.41739870290668,
-0.121817958968287));
#16154=CARTESIAN_POINT('Ctrl Pts',(0.384911758361269,-0.38663653976279,
-0.109029967924066));
#16155=CARTESIAN_POINT('Ctrl Pts',(0.38761064154154,-0.372652407310247,
-0.0994291026068839));
#16156=CARTESIAN_POINT('Ctrl Pts',(0.392612801026882,-0.350574799681989,
-0.0773514949786256));
#16157=CARTESIAN_POINT('Ctrl Pts',(0.395252954914593,-0.340970918840894,
-0.0633657881355917));
#16158=CARTESIAN_POINT('Ctrl Pts',(0.398970551469948,-0.328180693480621,
-0.0325978607437828));
#16159=CARTESIAN_POINT('Ctrl Pts',(0.4,-0.325,-0.0158075115832675));
#16160=CARTESIAN_POINT('Ctrl Pts',(0.4,-0.325,0.0158075115832676));
#16161=CARTESIAN_POINT('Ctrl Pts',(0.398970551469948,-0.328180693480621,
0.0325978607437829));
#16162=CARTESIAN_POINT('Ctrl Pts',(0.395252954914593,-0.340970918840894,
0.0633657881355918));
#16163=CARTESIAN_POINT('Ctrl Pts',(0.392612801026882,-0.350574799681989,
0.0773514949786257));
#16164=CARTESIAN_POINT('Ctrl Pts',(0.38761064154154,-0.372652407310247,
0.099429102606884));
#16165=CARTESIAN_POINT('Ctrl Pts',(0.384911758361269,-0.38663653976279,
0.109029967924066));
#16166=CARTESIAN_POINT('Ctrl Pts',(0.381057715344782,-0.41739870290668,
0.121817958968287));
#16167=CARTESIAN_POINT('Ctrl Pts',(0.379967103839267,-0.434186899370797,
0.125));
#16168=CARTESIAN_POINT('Ctrl Pts',(0.379967103839267,-0.45,0.125));
#16169=CARTESIAN_POINT('Ctrl Pts',(0.379967103839267,-0.45,0.125));
#16170=CARTESIAN_POINT('Ctrl Pts',(0.379967103839267,-0.465813100629203,
0.125));
#16171=CARTESIAN_POINT('Ctrl Pts',(0.381057715344782,-0.48260129709332,
0.121817958968287));
#16172=CARTESIAN_POINT('Ctrl Pts',(0.384911758361269,-0.51336346023721,
0.109029967924066));
#16173=CARTESIAN_POINT('Ctrl Pts',(0.38761064154154,-0.527347592689753,
0.0994291026068839));
#16174=CARTESIAN_POINT('Ctrl Pts',(0.392612801026882,-0.549425200318011,
0.0773514949786257));
#16175=CARTESIAN_POINT('Ctrl Pts',(0.395252954914593,-0.559029081159106,
0.0633657881355918));
#16176=CARTESIAN_POINT('Ctrl Pts',(0.398970551469948,-0.571819306519379,
0.0325978607437829));
#16177=CARTESIAN_POINT('Ctrl Pts',(0.4,-0.575,0.0158075115832676));
#16178=CARTESIAN_POINT('Ctrl Pts',(0.4,-0.575,-0.0158075115832676));
#16179=CARTESIAN_POINT('Ctrl Pts',(0.398970551469948,-0.57181930651938,
-0.0325978607437828));
#16180=CARTESIAN_POINT('Ctrl Pts',(0.395252954914593,-0.559029081159106,
-0.0633657881355918));
#16181=CARTESIAN_POINT('Ctrl Pts',(0.392612801026882,-0.549425200318011,
-0.0773514949786257));
#16182=CARTESIAN_POINT('Ctrl Pts',(0.38761064154154,-0.527347592689753,
-0.0994291026068839));
#16183=CARTESIAN_POINT('Ctrl Pts',(0.384911758361269,-0.51336346023721,
-0.109029967924066));
#16184=CARTESIAN_POINT('Ctrl Pts',(0.381057715344782,-0.48260129709332,
-0.121817958968287));
#16185=CARTESIAN_POINT('Ctrl Pts',(0.379967103839267,-0.465813100629203,
-0.125));
#16186=CARTESIAN_POINT('Ctrl Pts',(0.379967103839267,-0.45,-0.125));
#16187=CARTESIAN_POINT('',(0.637867541108654,-0.45,0.125));
#16188=CARTESIAN_POINT('',(-7.65404249467096E-18,-0.45,0.125));
#16189=CARTESIAN_POINT('',(0.65,-0.575,3.9801020972289E-17));
#16190=CARTESIAN_POINT('Ctrl Pts',(0.65,-0.575,5.55111512312578E-17));
#16191=CARTESIAN_POINT('Ctrl Pts',(0.65,-0.575,0.0157371373481999));
#16192=CARTESIAN_POINT('Ctrl Pts',(0.649370620646074,-0.571846918937749,
0.0324967135411165));
#16193=CARTESIAN_POINT('Ctrl Pts',(0.647096224417991,-0.559077918077178,
0.0632828231545124));
#16194=CARTESIAN_POINT('Ctrl Pts',(0.645482573914132,-0.549464140887802,
0.077312554408835));
#16195=CARTESIAN_POINT('Ctrl Pts',(0.642442040715078,-0.527312025401873,
0.099464669894764));
#16196=CARTESIAN_POINT('Ctrl Pts',(0.640815160902589,-0.513282519396725,
0.109078032552995));
#16197=CARTESIAN_POINT('Ctrl Pts',(0.63851034608138,-0.482497190457637,
0.121846732641678));
#16198=CARTESIAN_POINT('Ctrl Pts',(0.637867541108654,-0.465737888992352,
0.125));
#16199=CARTESIAN_POINT('Ctrl Pts',(0.637867541108654,-0.45,0.125));
#16200=CARTESIAN_POINT('',(0.65,-0.325,3.9801020972289E-17));
#16201=CARTESIAN_POINT('Ctrl Pts',(0.65,-0.325,6.93889390390723E-18));
#16202=CARTESIAN_POINT('Ctrl Pts',(0.65,-0.325,-0.0157371373481998));
#16203=CARTESIAN_POINT('Ctrl Pts',(0.649370620646074,-0.328153081062251,
-0.0324967135411164));
#16204=CARTESIAN_POINT('Ctrl Pts',(0.647096224417991,-0.340922081922822,
-0.0632828231545123));
#16205=CARTESIAN_POINT('Ctrl Pts',(0.645482573914132,-0.350535859112198,
-0.0773125544088349));
#16206=CARTESIAN_POINT('Ctrl Pts',(0.642442040715078,-0.372687974598127,
-0.0994646698947639));
#16207=CARTESIAN_POINT('Ctrl Pts',(0.640815160902588,-0.386717480603275,
-0.109078032552995));
#16208=CARTESIAN_POINT('Ctrl Pts',(0.63851034608138,-0.417502809542363,
-0.121846732641678));
#16209=CARTESIAN_POINT('Ctrl Pts',(0.637867541108654,-0.434262111007648,
-0.125));
#16210=CARTESIAN_POINT('Ctrl Pts',(0.637867541108654,-0.465737888992352,
-0.125));
#16211=CARTESIAN_POINT('Ctrl Pts',(0.63851034608138,-0.482497190457637,
-0.121846732641678));
#16212=CARTESIAN_POINT('Ctrl Pts',(0.640815160902589,-0.513282519396725,
-0.109078032552995));
#16213=CARTESIAN_POINT('Ctrl Pts',(0.642442040715078,-0.527312025401873,
-0.0994646698947639));
#16214=CARTESIAN_POINT('Ctrl Pts',(0.645482573914132,-0.549464140887802,
-0.0773125544088348));
#16215=CARTESIAN_POINT('Ctrl Pts',(0.647096224417991,-0.559077918077178,
-0.0632828231545123));
#16216=CARTESIAN_POINT('Ctrl Pts',(0.649370620646074,-0.571846918937749,
-0.0324967135411164));
#16217=CARTESIAN_POINT('Ctrl Pts',(0.65,-0.575,-0.0157371373481998));
#16218=CARTESIAN_POINT('Ctrl Pts',(0.65,-0.575,6.24500451351651E-17));
#16219=CARTESIAN_POINT('Ctrl Pts',(0.637867541108654,-0.45,0.125));
#16220=CARTESIAN_POINT('Ctrl Pts',(0.637867541108654,-0.434262111007648,
0.125));
#16221=CARTESIAN_POINT('Ctrl Pts',(0.63851034608138,-0.417502809542363,
0.121846732641678));
#16222=CARTESIAN_POINT('Ctrl Pts',(0.640815160902589,-0.386717480603274,
0.109078032552995));
#16223=CARTESIAN_POINT('Ctrl Pts',(0.642442040715078,-0.372687974598127,
0.0994646698947639));
#16224=CARTESIAN_POINT('Ctrl Pts',(0.645482573914132,-0.350535859112198,
0.0773125544088348));
#16225=CARTESIAN_POINT('Ctrl Pts',(0.647096224417991,-0.340922081922822,
0.0632828231545123));
#16226=CARTESIAN_POINT('Ctrl Pts',(0.649370620646074,-0.328153081062251,
0.0324967135411164));
#16227=CARTESIAN_POINT('Ctrl Pts',(0.65,-0.325,0.0157371373481998));
#16228=CARTESIAN_POINT('Ctrl Pts',(0.65,-0.325,-6.93889390390723E-18));
#16229=CARTESIAN_POINT('Origin',(0.,-0.1,0.));
#16230=CARTESIAN_POINT('',(-0.65,-0.8,7.9602041944578E-17));
#16231=CARTESIAN_POINT('Origin',(0.,-0.8,0.));
#16232=CARTESIAN_POINT('',(-0.65,-0.1,-7.9602041944578E-17));
#16233=CARTESIAN_POINT('',(-0.65,-0.1,7.9602041944578E-17));
#16234=CARTESIAN_POINT('',(-0.65,-0.1,-7.9602041944578E-17));
#16235=CARTESIAN_POINT('Origin',(0.,-0.1,0.));
#16236=CARTESIAN_POINT('',(0.,-0.575,-0.65));
#16237=CARTESIAN_POINT('',(0.,-0.325,-0.65));
#16238=CARTESIAN_POINT('Ctrl Pts',(-1.73472347597681E-17,-0.575,-0.65));
#16239=CARTESIAN_POINT('Ctrl Pts',(0.0157371373481998,-0.575,-0.65));
#16240=CARTESIAN_POINT('Ctrl Pts',(0.0324967135411164,-0.571846918937749,
-0.649370620646074));
#16241=CARTESIAN_POINT('Ctrl Pts',(0.0632828231545123,-0.559077918077178,
-0.647096224417991));
#16242=CARTESIAN_POINT('Ctrl Pts',(0.0773125544088349,-0.549464140887802,
-0.645482573914132));
#16243=CARTESIAN_POINT('Ctrl Pts',(0.099464669894764,-0.527312025401873,
-0.642442040715078));
#16244=CARTESIAN_POINT('Ctrl Pts',(0.109078032552995,-0.513282519396725,
-0.640815160902589));
#16245=CARTESIAN_POINT('Ctrl Pts',(0.121846732641678,-0.482497190457636,
-0.63851034608138));
#16246=CARTESIAN_POINT('Ctrl Pts',(0.125,-0.465737888992352,-0.637867541108654));
#16247=CARTESIAN_POINT('Ctrl Pts',(0.125,-0.434262111007648,-0.637867541108654));
#16248=CARTESIAN_POINT('Ctrl Pts',(0.121846732641678,-0.417502809542364,
-0.63851034608138));
#16249=CARTESIAN_POINT('Ctrl Pts',(0.109078032552995,-0.386717480603275,
-0.640815160902589));
#16250=CARTESIAN_POINT('Ctrl Pts',(0.099464669894764,-0.372687974598127,
-0.642442040715078));
#16251=CARTESIAN_POINT('Ctrl Pts',(0.0773125544088349,-0.350535859112198,
-0.645482573914132));
#16252=CARTESIAN_POINT('Ctrl Pts',(0.0632828231545123,-0.340922081922822,
-0.647096224417991));
#16253=CARTESIAN_POINT('Ctrl Pts',(0.0324967135411164,-0.328153081062251,
-0.649370620646074));
#16254=CARTESIAN_POINT('Ctrl Pts',(0.0157371373481999,-0.325,-0.65));
#16255=CARTESIAN_POINT('Ctrl Pts',(4.5102810375397E-17,-0.325,-0.65));
#16256=CARTESIAN_POINT('',(-0.125,-0.45,-0.637867541108654));
#16257=CARTESIAN_POINT('Ctrl Pts',(4.85722573273506E-17,-0.325,-0.65));
#16258=CARTESIAN_POINT('Ctrl Pts',(-0.0157371373481997,-0.325,-0.65));
#16259=CARTESIAN_POINT('Ctrl Pts',(-0.0324967135411163,-0.328153081062251,
-0.649370620646074));
#16260=CARTESIAN_POINT('Ctrl Pts',(-0.0632828231545122,-0.340922081922822,
-0.647096224417991));
#16261=CARTESIAN_POINT('Ctrl Pts',(-0.0773125544088348,-0.350535859112198,
-0.645482573914132));
#16262=CARTESIAN_POINT('Ctrl Pts',(-0.0994646698947639,-0.372687974598127,
-0.642442040715078));
#16263=CARTESIAN_POINT('Ctrl Pts',(-0.109078032552995,-0.386717480603274,
-0.640815160902589));
#16264=CARTESIAN_POINT('Ctrl Pts',(-0.121846732641678,-0.417502809542363,
-0.63851034608138));
#16265=CARTESIAN_POINT('Ctrl Pts',(-0.125,-0.434262111007648,-0.637867541108654));
#16266=CARTESIAN_POINT('Ctrl Pts',(-0.125,-0.45,-0.637867541108654));
#16267=CARTESIAN_POINT('Ctrl Pts',(-0.125,-0.45,-0.637867541108654));
#16268=CARTESIAN_POINT('Ctrl Pts',(-0.125,-0.465737888992352,-0.637867541108654));
#16269=CARTESIAN_POINT('Ctrl Pts',(-0.121846732641678,-0.482497190457636,
-0.63851034608138));
#16270=CARTESIAN_POINT('Ctrl Pts',(-0.109078032552995,-0.513282519396725,
-0.640815160902589));
#16271=CARTESIAN_POINT('Ctrl Pts',(-0.099464669894764,-0.527312025401873,
-0.642442040715078));
#16272=CARTESIAN_POINT('Ctrl Pts',(-0.0773125544088349,-0.549464140887802,
-0.645482573914132));
#16273=CARTESIAN_POINT('Ctrl Pts',(-0.0632828231545124,-0.559077918077178,
-0.647096224417991));
#16274=CARTESIAN_POINT('Ctrl Pts',(-0.0324967135411165,-0.571846918937749,
-0.649370620646074));
#16275=CARTESIAN_POINT('Ctrl Pts',(-0.0157371373481998,-0.575,-0.65));
#16276=CARTESIAN_POINT('Ctrl Pts',(-1.73472347597681E-17,-0.575,-0.65));
#16277=CARTESIAN_POINT('',(0.,-0.325,0.65));
#16278=CARTESIAN_POINT('',(0.,-0.575,0.65));
#16279=CARTESIAN_POINT('Ctrl Pts',(2.77555756156289E-17,-0.325,0.65));
#16280=CARTESIAN_POINT('Ctrl Pts',(0.0157371373481998,-0.325,0.65));
#16281=CARTESIAN_POINT('Ctrl Pts',(0.0324967135411164,-0.328153081062251,
0.649370620646074));
#16282=CARTESIAN_POINT('Ctrl Pts',(0.0632828231545123,-0.340922081922822,
0.647096224417991));
#16283=CARTESIAN_POINT('Ctrl Pts',(0.0773125544088349,-0.350535859112198,
0.645482573914132));
#16284=CARTESIAN_POINT('Ctrl Pts',(0.099464669894764,-0.372687974598127,
0.642442040715078));
#16285=CARTESIAN_POINT('Ctrl Pts',(0.109078032552995,-0.386717480603275,
0.640815160902589));
#16286=CARTESIAN_POINT('Ctrl Pts',(0.121846732641678,-0.417502809542364,
0.63851034608138));
#16287=CARTESIAN_POINT('Ctrl Pts',(0.125,-0.434262111007648,0.637867541108654));
#16288=CARTESIAN_POINT('Ctrl Pts',(0.125,-0.465737888992352,0.637867541108654));
#16289=CARTESIAN_POINT('Ctrl Pts',(0.121846732641678,-0.482497190457636,
0.63851034608138));
#16290=CARTESIAN_POINT('Ctrl Pts',(0.109078032552995,-0.513282519396725,
0.640815160902589));
#16291=CARTESIAN_POINT('Ctrl Pts',(0.099464669894764,-0.527312025401873,
0.642442040715078));
#16292=CARTESIAN_POINT('Ctrl Pts',(0.077312554408835,-0.549464140887802,
0.645482573914132));
#16293=CARTESIAN_POINT('Ctrl Pts',(0.0632828231545124,-0.559077918077178,
0.647096224417991));
#16294=CARTESIAN_POINT('Ctrl Pts',(0.0324967135411165,-0.571846918937749,
0.649370620646074));
#16295=CARTESIAN_POINT('Ctrl Pts',(0.0157371373481998,-0.575,0.65));
#16296=CARTESIAN_POINT('Ctrl Pts',(-1.38777878078145E-17,-0.575,0.65));
#16297=CARTESIAN_POINT('',(-0.125,-0.45,0.637867541108654));
#16298=CARTESIAN_POINT('Ctrl Pts',(-1.04083408558608E-17,-0.575,0.65));
#16299=CARTESIAN_POINT('Ctrl Pts',(-0.0157371373481998,-0.575,0.65));
#16300=CARTESIAN_POINT('Ctrl Pts',(-0.0324967135411164,-0.571846918937749,
0.649370620646074));
#16301=CARTESIAN_POINT('Ctrl Pts',(-0.0632828231545123,-0.559077918077178,
0.647096224417991));
#16302=CARTESIAN_POINT('Ctrl Pts',(-0.0773125544088349,-0.549464140887802,
0.645482573914132));
#16303=CARTESIAN_POINT('Ctrl Pts',(-0.099464669894764,-0.527312025401873,
0.642442040715078));
#16304=CARTESIAN_POINT('Ctrl Pts',(-0.109078032552995,-0.513282519396725,
0.640815160902589));
#16305=CARTESIAN_POINT('Ctrl Pts',(-0.121846732641678,-0.482497190457636,
0.63851034608138));
#16306=CARTESIAN_POINT('Ctrl Pts',(-0.125,-0.465737888992352,0.637867541108654));
#16307=CARTESIAN_POINT('Ctrl Pts',(-0.125,-0.45,0.637867541108654));
#16308=CARTESIAN_POINT('Ctrl Pts',(-0.125,-0.45,0.637867541108654));
#16309=CARTESIAN_POINT('Ctrl Pts',(-0.125,-0.434262111007648,0.637867541108654));
#16310=CARTESIAN_POINT('Ctrl Pts',(-0.121846732641678,-0.417502809542363,
0.63851034608138));
#16311=CARTESIAN_POINT('Ctrl Pts',(-0.109078032552995,-0.386717480603274,
0.640815160902589));
#16312=CARTESIAN_POINT('Ctrl Pts',(-0.0994646698947639,-0.372687974598127,
0.642442040715078));
#16313=CARTESIAN_POINT('Ctrl Pts',(-0.0773125544088348,-0.350535859112198,
0.645482573914132));
#16314=CARTESIAN_POINT('Ctrl Pts',(-0.0632828231545122,-0.340922081922822,
0.647096224417991));
#16315=CARTESIAN_POINT('Ctrl Pts',(-0.0324967135411163,-0.328153081062251,
0.649370620646074));
#16316=CARTESIAN_POINT('Ctrl Pts',(-0.0157371373481998,-0.325,0.65));
#16317=CARTESIAN_POINT('Ctrl Pts',(4.5102810375397E-17,-0.325,0.65));
#16318=CARTESIAN_POINT('Origin',(0.,-0.45,0.));
#16319=CARTESIAN_POINT('',(-0.125,-0.45,-0.379967103839267));
#16320=CARTESIAN_POINT('',(-0.125,-0.45,0.));
#16321=CARTESIAN_POINT('',(0.125,-0.45,-0.379967103839267));
#16322=CARTESIAN_POINT('Ctrl Pts',(0.125,-0.45,-0.379967103839267));
#16323=CARTESIAN_POINT('Ctrl Pts',(0.125,-0.465813100629203,-0.379967103839267));
#16324=CARTESIAN_POINT('Ctrl Pts',(0.121817958968287,-0.48260129709332,
-0.381057715344782));
#16325=CARTESIAN_POINT('Ctrl Pts',(0.109029967924066,-0.51336346023721,
-0.384911758361269));
#16326=CARTESIAN_POINT('Ctrl Pts',(0.0994291026068839,-0.527347592689753,
-0.38761064154154));
#16327=CARTESIAN_POINT('Ctrl Pts',(0.0773514949786257,-0.549425200318011,
-0.392612801026882));
#16328=CARTESIAN_POINT('Ctrl Pts',(0.0633657881355918,-0.559029081159106,
-0.395252954914593));
#16329=CARTESIAN_POINT('Ctrl Pts',(0.0325978607437828,-0.571819306519379,
-0.398970551469948));
#16330=CARTESIAN_POINT('Ctrl Pts',(0.0158075115832676,-0.575,-0.4));
#16331=CARTESIAN_POINT('Ctrl Pts',(-0.0158075115832676,-0.575,-0.4));
#16332=CARTESIAN_POINT('Ctrl Pts',(-0.0325978607437828,-0.571819306519379,
-0.398970551469948));
#16333=CARTESIAN_POINT('Ctrl Pts',(-0.0633657881355918,-0.559029081159106,
-0.395252954914593));
#16334=CARTESIAN_POINT('Ctrl Pts',(-0.0773514949786256,-0.549425200318011,
-0.392612801026882));
#16335=CARTESIAN_POINT('Ctrl Pts',(-0.0994291026068839,-0.527347592689753,
-0.38761064154154));
#16336=CARTESIAN_POINT('Ctrl Pts',(-0.109029967924066,-0.51336346023721,
-0.384911758361269));
#16337=CARTESIAN_POINT('Ctrl Pts',(-0.121817958968287,-0.48260129709332,
-0.381057715344782));
#16338=CARTESIAN_POINT('Ctrl Pts',(-0.125,-0.465813100629203,-0.379967103839267));
#16339=CARTESIAN_POINT('Ctrl Pts',(-0.125,-0.45,-0.379967103839267));
#16340=CARTESIAN_POINT('Ctrl Pts',(-0.125,-0.45,-0.379967103839267));
#16341=CARTESIAN_POINT('Ctrl Pts',(-0.125,-0.434186899370797,-0.379967103839267));
#16342=CARTESIAN_POINT('Ctrl Pts',(-0.121817958968287,-0.41739870290668,
-0.381057715344782));
#16343=CARTESIAN_POINT('Ctrl Pts',(-0.109029967924066,-0.38663653976279,
-0.384911758361269));
#16344=CARTESIAN_POINT('Ctrl Pts',(-0.0994291026068839,-0.372652407310247,
-0.38761064154154));
#16345=CARTESIAN_POINT('Ctrl Pts',(-0.0773514949786257,-0.350574799681989,
-0.392612801026882));
#16346=CARTESIAN_POINT('Ctrl Pts',(-0.0633657881355918,-0.340970918840894,
-0.395252954914593));
#16347=CARTESIAN_POINT('Ctrl Pts',(-0.0325978607437829,-0.328180693480621,
-0.398970551469948));
#16348=CARTESIAN_POINT('Ctrl Pts',(-0.0158075115832676,-0.325,-0.4));
#16349=CARTESIAN_POINT('Ctrl Pts',(0.0158075115832675,-0.325,-0.4));
#16350=CARTESIAN_POINT('Ctrl Pts',(0.0325978607437828,-0.328180693480621,
-0.398970551469948));
#16351=CARTESIAN_POINT('Ctrl Pts',(0.0633657881355917,-0.340970918840894,
-0.395252954914593));
#16352=CARTESIAN_POINT('Ctrl Pts',(0.0773514949786256,-0.350574799681989,
-0.392612801026882));
#16353=CARTESIAN_POINT('Ctrl Pts',(0.0994291026068839,-0.372652407310247,
-0.38761064154154));
#16354=CARTESIAN_POINT('Ctrl Pts',(0.109029967924066,-0.38663653976279,
-0.384911758361269));
#16355=CARTESIAN_POINT('Ctrl Pts',(0.121817958968287,-0.41739870290668,
-0.381057715344782));
#16356=CARTESIAN_POINT('Ctrl Pts',(0.125,-0.434186899370797,-0.379967103839267));
#16357=CARTESIAN_POINT('Ctrl Pts',(0.125,-0.45,-0.379967103839267));
#16358=CARTESIAN_POINT('Origin',(0.,-0.45,0.));
#16359=CARTESIAN_POINT('',(0.125,-0.45,0.379967103839267));
#16360=CARTESIAN_POINT('',(-0.125,-0.45,0.379967103839267));
#16361=CARTESIAN_POINT('Ctrl Pts',(0.125,-0.45,0.379967103839267));
#16362=CARTESIAN_POINT('Ctrl Pts',(0.125,-0.434186899370797,0.379967103839267));
#16363=CARTESIAN_POINT('Ctrl Pts',(0.121817958968287,-0.41739870290668,
0.381057715344782));
#16364=CARTESIAN_POINT('Ctrl Pts',(0.109029967924066,-0.38663653976279,
0.384911758361269));
#16365=CARTESIAN_POINT('Ctrl Pts',(0.0994291026068839,-0.372652407310247,
0.38761064154154));
#16366=CARTESIAN_POINT('Ctrl Pts',(0.0773514949786256,-0.350574799681989,
0.392612801026882));
#16367=CARTESIAN_POINT('Ctrl Pts',(0.0633657881355918,-0.340970918840894,
0.395252954914593));
#16368=CARTESIAN_POINT('Ctrl Pts',(0.0325978607437828,-0.328180693480621,
0.398970551469948));
#16369=CARTESIAN_POINT('Ctrl Pts',(0.0158075115832676,-0.325,0.4));
#16370=CARTESIAN_POINT('Ctrl Pts',(-0.0158075115832676,-0.325,0.4));
#16371=CARTESIAN_POINT('Ctrl Pts',(-0.0325978607437828,-0.328180693480621,
0.398970551469948));
#16372=CARTESIAN_POINT('Ctrl Pts',(-0.0633657881355918,-0.340970918840894,
0.395252954914593));
#16373=CARTESIAN_POINT('Ctrl Pts',(-0.0773514949786257,-0.350574799681989,
0.392612801026882));
#16374=CARTESIAN_POINT('Ctrl Pts',(-0.0994291026068839,-0.372652407310247,
0.38761064154154));
#16375=CARTESIAN_POINT('Ctrl Pts',(-0.109029967924066,-0.38663653976279,
0.384911758361269));
#16376=CARTESIAN_POINT('Ctrl Pts',(-0.121817958968287,-0.41739870290668,
0.381057715344782));
#16377=CARTESIAN_POINT('Ctrl Pts',(-0.125,-0.434186899370797,0.379967103839267));
#16378=CARTESIAN_POINT('Ctrl Pts',(-0.125,-0.45,0.379967103839267));
#16379=CARTESIAN_POINT('Ctrl Pts',(-0.125,-0.45,0.379967103839267));
#16380=CARTESIAN_POINT('Ctrl Pts',(-0.125,-0.465813100629203,0.379967103839267));
#16381=CARTESIAN_POINT('Ctrl Pts',(-0.121817958968287,-0.48260129709332,
0.381057715344782));
#16382=CARTESIAN_POINT('Ctrl Pts',(-0.109029967924066,-0.51336346023721,
0.384911758361269));
#16383=CARTESIAN_POINT('Ctrl Pts',(-0.0994291026068839,-0.527347592689753,
0.38761064154154));
#16384=CARTESIAN_POINT('Ctrl Pts',(-0.0773514949786256,-0.549425200318011,
0.392612801026882));
#16385=CARTESIAN_POINT('Ctrl Pts',(-0.0633657881355917,-0.559029081159106,
0.395252954914593));
#16386=CARTESIAN_POINT('Ctrl Pts',(-0.0325978607437828,-0.571819306519379,
0.398970551469948));
#16387=CARTESIAN_POINT('Ctrl Pts',(-0.0158075115832675,-0.575,0.4));
#16388=CARTESIAN_POINT('Ctrl Pts',(0.0158075115832676,-0.575,0.4));
#16389=CARTESIAN_POINT('Ctrl Pts',(0.0325978607437828,-0.571819306519379,
0.398970551469948));
#16390=CARTESIAN_POINT('Ctrl Pts',(0.0633657881355917,-0.559029081159106,
0.395252954914593));
#16391=CARTESIAN_POINT('Ctrl Pts',(0.0773514949786257,-0.549425200318011,
0.392612801026882));
#16392=CARTESIAN_POINT('Ctrl Pts',(0.0994291026068839,-0.527347592689753,
0.38761064154154));
#16393=CARTESIAN_POINT('Ctrl Pts',(0.109029967924066,-0.51336346023721,
0.384911758361269));
#16394=CARTESIAN_POINT('Ctrl Pts',(0.121817958968287,-0.48260129709332,
0.381057715344782));
#16395=CARTESIAN_POINT('Ctrl Pts',(0.125,-0.465813100629203,0.379967103839267));
#16396=CARTESIAN_POINT('Ctrl Pts',(0.125,-0.45,0.379967103839267));
#16397=CARTESIAN_POINT('',(-0.125,-0.45,0.));
#16398=CARTESIAN_POINT('Origin',(0.,0.,0.));
#16399=CARTESIAN_POINT('',(-0.4,-0.8,4.89858719658941E-17));
#16400=CARTESIAN_POINT('Origin',(0.,-0.8,0.));
#16401=CARTESIAN_POINT('',(-0.4,0.,4.89858719658941E-17));
#16402=CARTESIAN_POINT('',(-0.4,0.85,-4.89858719658941E-17));
#16403=CARTESIAN_POINT('',(-0.4,0.,4.89858719658941E-17));
#16404=CARTESIAN_POINT('Origin',(0.,0.85,0.));
#16405=CARTESIAN_POINT('Origin',(0.,-0.8,0.));
#16406=CARTESIAN_POINT('Origin',(0.,0.,0.));
#16407=CARTESIAN_POINT('',(-0.8,0.,9.79717439317883E-17));
#16408=CARTESIAN_POINT('Origin',(0.,0.,0.));
#16409=CARTESIAN_POINT('',(0.595438916863769,0.,0.137993139022126));
#16410=CARTESIAN_POINT('',(0.562830534889751,0.,0.238351419397483));
#16411=CARTESIAN_POINT('Origin',(0.562758945330873,0.,0.182851465569258));
#16412=CARTESIAN_POINT('',(0.523653836874034,0.,0.315240018494132));
#16413=CARTESIAN_POINT('Origin',(0.,0.,0.));
#16414=CARTESIAN_POINT('',(0.461629008549572,0.,0.40060987082025));
#16415=CARTESIAN_POINT('Origin',(0.478711351753049,0.,0.347804155687524));
#16416=CARTESIAN_POINT('',(0.40060987082025,0.,0.461629008549572));
#16417=CARTESIAN_POINT('Origin',(0.,0.,0.));
#16418=CARTESIAN_POINT('',(0.315240018494132,0.,0.523653836874034));
#16419=CARTESIAN_POINT('Origin',(0.347804155687523,0.,0.478711351753049));
#16420=CARTESIAN_POINT('',(0.238351419397483,0.,0.562830534889751));
#16421=CARTESIAN_POINT('Origin',(0.,0.,0.));
#16422=CARTESIAN_POINT('',(0.137993139022126,0.,0.595438916863769));
#16423=CARTESIAN_POINT('Origin',(0.182851465569258,0.,0.562758945330873));
#16424=CARTESIAN_POINT('',(0.0527614703521001,0.,0.608938287003997));
#16425=CARTESIAN_POINT('Origin',(0.,0.,0.));
#16426=CARTESIAN_POINT('',(-0.0527614703521003,0.,0.608938287003997));
#16427=CARTESIAN_POINT('Origin',(-1.08697158783324E-16,0.,0.591719772367581));
#16428=CARTESIAN_POINT('',(-0.137993139022126,0.,0.595438916863769));
#16429=CARTESIAN_POINT('Origin',(0.,0.,0.));
#16430=CARTESIAN_POINT('',(-0.238351419397483,0.,0.562830534889751));
#16431=CARTESIAN_POINT('Origin',(-0.182851465569258,0.,0.562758945330873));
#16432=CARTESIAN_POINT('',(-0.315240018494132,0.,0.523653836874034));
#16433=CARTESIAN_POINT('Origin',(0.,0.,0.));
#16434=CARTESIAN_POINT('',(-0.40060987082025,0.,0.461629008549572));
#16435=CARTESIAN_POINT('Origin',(-0.347804155687524,0.,0.478711351753049));
#16436=CARTESIAN_POINT('',(-0.461629008549572,0.,0.40060987082025));
#16437=CARTESIAN_POINT('Origin',(0.,0.,0.));
#16438=CARTESIAN_POINT('',(-0.523653836874034,0.,0.315240018494132));
#16439=CARTESIAN_POINT('Origin',(-0.478711351753049,0.,0.347804155687524));
#16440=CARTESIAN_POINT('',(-0.562830534889751,0.,0.238351419397483));
#16441=CARTESIAN_POINT('Origin',(0.,0.,0.));
#16442=CARTESIAN_POINT('',(-0.595438916863769,0.,0.137993139022126));
#16443=CARTESIAN_POINT('Origin',(-0.562758945330873,0.,0.182851465569258));
#16444=CARTESIAN_POINT('',(-0.608938287003997,0.,0.0527614703521002));
#16445=CARTESIAN_POINT('Origin',(0.,0.,0.));
#16446=CARTESIAN_POINT('',(-0.608938287003997,0.,-0.0527614703521003));
#16447=CARTESIAN_POINT('Origin',(-0.591719772367581,0.,-7.24647725222159E-17));
#16448=CARTESIAN_POINT('',(-0.595438916863769,0.,-0.137993139022126));
#16449=CARTESIAN_POINT('Origin',(0.,0.,0.));
#16450=CARTESIAN_POINT('',(-0.562830534889751,0.,-0.238351419397483));
#16451=CARTESIAN_POINT('Origin',(-0.562758945330873,0.,-0.182851465569258));
#16452=CARTESIAN_POINT('',(-0.523653836874034,0.,-0.315240018494132));
#16453=CARTESIAN_POINT('Origin',(0.,0.,0.));
#16454=CARTESIAN_POINT('',(-0.461629008549572,0.,-0.40060987082025));
#16455=CARTESIAN_POINT('Origin',(-0.478711351753049,0.,-0.347804155687524));
#16456=CARTESIAN_POINT('',(-0.40060987082025,0.,-0.461629008549572));
#16457=CARTESIAN_POINT('Origin',(0.,0.,0.));
#16458=CARTESIAN_POINT('',(-0.315240018494132,0.,-0.523653836874034));
#16459=CARTESIAN_POINT('Origin',(-0.347804155687524,0.,-0.478711351753049));
#16460=CARTESIAN_POINT('',(-0.238351419397483,0.,-0.562830534889751));
#16461=CARTESIAN_POINT('Origin',(0.,0.,0.));
#16462=CARTESIAN_POINT('',(-0.137993139022126,0.,-0.595438916863769));
#16463=CARTESIAN_POINT('Origin',(-0.182851465569258,0.,-0.562758945330873));
#16464=CARTESIAN_POINT('',(-0.0527614703521002,0.,-0.608938287003997));
#16465=CARTESIAN_POINT('Origin',(0.,0.,0.));
#16466=CARTESIAN_POINT('',(0.0527614703521003,0.,-0.608938287003997));
#16467=CARTESIAN_POINT('Origin',(3.6232386261108E-17,0.,-0.591719772367581));
#16468=CARTESIAN_POINT('',(0.137993139022126,0.,-0.595438916863769));
#16469=CARTESIAN_POINT('Origin',(0.,0.,0.));
#16470=CARTESIAN_POINT('',(0.238351419397483,0.,-0.562830534889751));
#16471=CARTESIAN_POINT('Origin',(0.182851465569258,0.,-0.562758945330873));
#16472=CARTESIAN_POINT('',(0.315240018494132,0.,-0.523653836874034));
#16473=CARTESIAN_POINT('Origin',(0.,0.,0.));
#16474=CARTESIAN_POINT('',(0.40060987082025,0.,-0.461629008549572));
#16475=CARTESIAN_POINT('Origin',(0.347804155687524,0.,-0.478711351753049));
#16476=CARTESIAN_POINT('',(0.461629008549572,0.,-0.40060987082025));
#16477=CARTESIAN_POINT('Origin',(0.,0.,0.));
#16478=CARTESIAN_POINT('',(0.523653836874034,0.,-0.315240018494132));
#16479=CARTESIAN_POINT('Origin',(0.478711351753049,0.,-0.347804155687524));
#16480=CARTESIAN_POINT('',(0.562830534889751,0.,-0.238351419397483));
#16481=CARTESIAN_POINT('Origin',(0.,0.,0.));
#16482=CARTESIAN_POINT('',(0.595438916863769,0.,-0.137993139022126));
#16483=CARTESIAN_POINT('Origin',(0.562758945330873,0.,-0.182851465569258));
#16484=CARTESIAN_POINT('',(0.608938287003997,0.,-0.0527614703521001));
#16485=CARTESIAN_POINT('Origin',(0.,0.,0.));
#16486=CARTESIAN_POINT('',(0.608938287003997,0.,0.0527614703521001));
#16487=CARTESIAN_POINT('Origin',(0.591719772367581,0.,0.));
#16488=CARTESIAN_POINT('Origin',(0.,0.,0.));
#16489=CARTESIAN_POINT('Origin',(0.,0.,0.));
#16490=CARTESIAN_POINT('',(-0.8,-0.1,9.79717439317883E-17));
#16491=CARTESIAN_POINT('Origin',(0.,-0.1,0.));
#16492=CARTESIAN_POINT('',(-0.8,0.,-9.79717439317883E-17));
#16493=CARTESIAN_POINT('Origin',(0.,-0.1,0.));
#16494=CARTESIAN_POINT('Origin',(0.,0.75,0.));
#16495=CARTESIAN_POINT('',(-0.8,0.75,9.79717439317883E-17));
#16496=CARTESIAN_POINT('Origin',(0.,0.75,0.));
#16497=CARTESIAN_POINT('',(0.562830534889751,0.75,0.238351419397483));
#16498=CARTESIAN_POINT('',(0.595438916863769,0.75,0.137993139022126));
#16499=CARTESIAN_POINT('Origin',(0.562758945330873,0.75,0.182851465569258));
#16500=CARTESIAN_POINT('',(0.608938287003997,0.75,0.0527614703521002));
#16501=CARTESIAN_POINT('Origin',(0.,0.75,0.));
#16502=CARTESIAN_POINT('',(0.608938287003997,0.75,-0.0527614703521002));
#16503=CARTESIAN_POINT('Origin',(0.591719772367581,0.75,0.));
#16504=CARTESIAN_POINT('',(0.595438916863769,0.75,-0.137993139022126));
#16505=CARTESIAN_POINT('Origin',(0.,0.75,0.));
#16506=CARTESIAN_POINT('',(0.562830534889751,0.75,-0.238351419397483));
#16507=CARTESIAN_POINT('Origin',(0.562758945330873,0.75,-0.182851465569258));
#16508=CARTESIAN_POINT('',(0.523653836874034,0.75,-0.315240018494132));
#16509=CARTESIAN_POINT('Origin',(0.,0.75,0.));
#16510=CARTESIAN_POINT('',(0.461629008549572,0.75,-0.40060987082025));
#16511=CARTESIAN_POINT('Origin',(0.478711351753049,0.75,-0.347804155687524));
#16512=CARTESIAN_POINT('',(0.40060987082025,0.75,-0.461629008549572));
#16513=CARTESIAN_POINT('Origin',(0.,0.75,0.));
#16514=CARTESIAN_POINT('',(0.315240018494132,0.75,-0.523653836874034));
#16515=CARTESIAN_POINT('Origin',(0.347804155687524,0.75,-0.478711351753049));
#16516=CARTESIAN_POINT('',(0.238351419397483,0.75,-0.562830534889751));
#16517=CARTESIAN_POINT('Origin',(0.,0.75,0.));
#16518=CARTESIAN_POINT('',(0.137993139022126,0.75,-0.595438916863769));
#16519=CARTESIAN_POINT('Origin',(0.182851465569258,0.75,-0.562758945330873));
#16520=CARTESIAN_POINT('',(0.0527614703521003,0.75,-0.608938287003997));
#16521=CARTESIAN_POINT('Origin',(0.,0.75,0.));
#16522=CARTESIAN_POINT('',(-0.0527614703521002,0.75,-0.608938287003997));
#16523=CARTESIAN_POINT('Origin',(3.6232386261108E-17,0.75,-0.591719772367581));
#16524=CARTESIAN_POINT('',(-0.137993139022126,0.75,-0.595438916863769));
#16525=CARTESIAN_POINT('Origin',(0.,0.75,0.));
#16526=CARTESIAN_POINT('',(-0.238351419397483,0.75,-0.562830534889751));
#16527=CARTESIAN_POINT('Origin',(-0.182851465569258,0.75,-0.562758945330873));
#16528=CARTESIAN_POINT('',(-0.315240018494132,0.75,-0.523653836874034));
#16529=CARTESIAN_POINT('Origin',(0.,0.75,0.));
#16530=CARTESIAN_POINT('',(-0.40060987082025,0.75,-0.461629008549572));
#16531=CARTESIAN_POINT('Origin',(-0.347804155687524,0.75,-0.478711351753049));
#16532=CARTESIAN_POINT('',(-0.461629008549572,0.75,-0.40060987082025));
#16533=CARTESIAN_POINT('Origin',(0.,0.75,0.));
#16534=CARTESIAN_POINT('',(-0.523653836874034,0.75,-0.315240018494132));
#16535=CARTESIAN_POINT('Origin',(-0.478711351753049,0.75,-0.347804155687524));
#16536=CARTESIAN_POINT('',(-0.562830534889751,0.75,-0.238351419397483));
#16537=CARTESIAN_POINT('Origin',(0.,0.75,0.));
#16538=CARTESIAN_POINT('',(-0.595438916863769,0.75,-0.137993139022126));
#16539=CARTESIAN_POINT('Origin',(-0.562758945330873,0.75,-0.182851465569258));
#16540=CARTESIAN_POINT('',(-0.608938287003997,0.75,-0.0527614703521003));
#16541=CARTESIAN_POINT('Origin',(0.,0.75,0.));
#16542=CARTESIAN_POINT('',(-0.608938287003997,0.75,0.0527614703521002));
#16543=CARTESIAN_POINT('Origin',(-0.591719772367581,0.75,-7.24647725222159E-17));
#16544=CARTESIAN_POINT('',(-0.595438916863769,0.75,0.137993139022126));
#16545=CARTESIAN_POINT('Origin',(0.,0.75,0.));
#16546=CARTESIAN_POINT('',(-0.562830534889751,0.75,0.238351419397483));
#16547=CARTESIAN_POINT('Origin',(-0.562758945330873,0.75,0.182851465569258));
#16548=CARTESIAN_POINT('',(-0.523653836874034,0.75,0.315240018494132));
#16549=CARTESIAN_POINT('Origin',(0.,0.75,0.));
#16550=CARTESIAN_POINT('',(-0.461629008549572,0.75,0.40060987082025));
#16551=CARTESIAN_POINT('Origin',(-0.478711351753049,0.75,0.347804155687524));
#16552=CARTESIAN_POINT('',(-0.40060987082025,0.75,0.461629008549572));
#16553=CARTESIAN_POINT('Origin',(0.,0.75,0.));
#16554=CARTESIAN_POINT('',(-0.315240018494132,0.75,0.523653836874034));
#16555=CARTESIAN_POINT('Origin',(-0.347804155687524,0.75,0.478711351753049));
#16556=CARTESIAN_POINT('',(-0.238351419397483,0.75,0.562830534889751));
#16557=CARTESIAN_POINT('Origin',(0.,0.75,0.));
#16558=CARTESIAN_POINT('',(-0.137993139022126,0.75,0.595438916863769));
#16559=CARTESIAN_POINT('Origin',(-0.182851465569258,0.75,0.562758945330873));
#16560=CARTESIAN_POINT('',(-0.0527614703521003,0.75,0.608938287003997));
#16561=CARTESIAN_POINT('Origin',(0.,0.75,0.));
#16562=CARTESIAN_POINT('',(0.0527614703521001,0.75,0.608938287003997));
#16563=CARTESIAN_POINT('Origin',(-1.08697158783324E-16,0.75,0.591719772367581));
#16564=CARTESIAN_POINT('',(0.137993139022126,0.75,0.595438916863769));
#16565=CARTESIAN_POINT('Origin',(0.,0.75,0.));
#16566=CARTESIAN_POINT('',(0.238351419397483,0.75,0.562830534889751));
#16567=CARTESIAN_POINT('Origin',(0.182851465569258,0.75,0.562758945330873));
#16568=CARTESIAN_POINT('',(0.315240018494132,0.75,0.523653836874034));
#16569=CARTESIAN_POINT('Origin',(0.,0.75,0.));
#16570=CARTESIAN_POINT('',(0.40060987082025,0.75,0.461629008549572));
#16571=CARTESIAN_POINT('Origin',(0.347804155687523,0.75,0.478711351753049));
#16572=CARTESIAN_POINT('',(0.461629008549572,0.75,0.40060987082025));
#16573=CARTESIAN_POINT('Origin',(0.,0.75,0.));
#16574=CARTESIAN_POINT('',(0.523653836874034,0.75,0.315240018494132));
#16575=CARTESIAN_POINT('Origin',(0.478711351753049,0.75,0.347804155687524));
#16576=CARTESIAN_POINT('Origin',(0.,0.75,0.));
#16577=CARTESIAN_POINT('Origin',(0.,0.75,0.));
#16578=CARTESIAN_POINT('',(-0.8,0.85,9.79717439317883E-17));
#16579=CARTESIAN_POINT('Origin',(0.,0.85,0.));
#16580=CARTESIAN_POINT('',(-0.8,0.75,9.79717439317883E-17));
#16581=CARTESIAN_POINT('Origin',(0.,0.85,0.));
#16582=CARTESIAN_POINT('Origin',(0.562758945330873,0.,0.182851465569258));
#16583=CARTESIAN_POINT('',(0.595438916863769,0.,0.137993139022126));
#16584=CARTESIAN_POINT('',(0.562830534889751,0.,0.238351419397483));
#16585=CARTESIAN_POINT('Origin',(0.,0.,0.));
#16586=CARTESIAN_POINT('',(0.523653836874034,0.,0.315240018494132));
#16587=CARTESIAN_POINT('Origin',(0.478711351753049,0.,0.347804155687524));
#16588=CARTESIAN_POINT('',(0.461629008549572,0.,0.40060987082025));
#16589=CARTESIAN_POINT('Origin',(0.,0.,0.));
#16590=CARTESIAN_POINT('',(0.40060987082025,0.,0.461629008549572));
#16591=CARTESIAN_POINT('Origin',(0.347804155687523,0.,0.478711351753049));
#16592=CARTESIAN_POINT('',(0.315240018494132,0.,0.523653836874034));
#16593=CARTESIAN_POINT('Origin',(0.,0.,0.));
#16594=CARTESIAN_POINT('',(0.238351419397483,0.,0.562830534889751));
#16595=CARTESIAN_POINT('Origin',(0.182851465569258,0.,0.562758945330873));
#16596=CARTESIAN_POINT('',(0.137993139022126,0.,0.595438916863769));
#16597=CARTESIAN_POINT('Origin',(0.,0.,0.));
#16598=CARTESIAN_POINT('',(0.0527614703521,0.,0.608938287003997));
#16599=CARTESIAN_POINT('Origin',(-1.08697158783324E-16,0.,0.591719772367581));
#16600=CARTESIAN_POINT('',(-0.0527614703521002,0.,0.608938287003997));
#16601=CARTESIAN_POINT('Origin',(0.,0.,0.));
#16602=CARTESIAN_POINT('',(-0.137993139022126,0.,0.595438916863769));
#16603=CARTESIAN_POINT('Origin',(-0.182851465569258,0.,0.562758945330873));
#16604=CARTESIAN_POINT('',(-0.238351419397483,0.,0.562830534889751));
#16605=CARTESIAN_POINT('Origin',(0.,0.,0.));
#16606=CARTESIAN_POINT('',(-0.315240018494132,0.,0.523653836874034));
#16607=CARTESIAN_POINT('Origin',(-0.347804155687524,0.,0.478711351753049));
#16608=CARTESIAN_POINT('',(-0.40060987082025,0.,0.461629008549572));
#16609=CARTESIAN_POINT('Origin',(0.,0.,0.));
#16610=CARTESIAN_POINT('',(-0.461629008549572,0.,0.40060987082025));
#16611=CARTESIAN_POINT('Origin',(-0.478711351753049,0.,0.347804155687524));
#16612=CARTESIAN_POINT('',(-0.523653836874034,0.,0.315240018494132));
#16613=CARTESIAN_POINT('Origin',(0.,0.,0.));
#16614=CARTESIAN_POINT('',(-0.562830534889751,0.,0.238351419397483));
#16615=CARTESIAN_POINT('Origin',(-0.562758945330873,0.,0.182851465569258));
#16616=CARTESIAN_POINT('',(-0.595438916863769,0.,0.137993139022126));
#16617=CARTESIAN_POINT('Origin',(0.,0.,0.));
#16618=CARTESIAN_POINT('',(-0.608938287003997,0.,0.0527614703521));
#16619=CARTESIAN_POINT('Origin',(-0.591719772367581,0.,-7.24647725222159E-17));
#16620=CARTESIAN_POINT('',(-0.608938287003997,0.,-0.0527614703521002));
#16621=CARTESIAN_POINT('Origin',(0.,0.,0.));
#16622=CARTESIAN_POINT('',(-0.595438916863769,0.,-0.137993139022126));
#16623=CARTESIAN_POINT('Origin',(-0.562758945330873,0.,-0.182851465569258));
#16624=CARTESIAN_POINT('',(-0.562830534889751,0.,-0.238351419397483));
#16625=CARTESIAN_POINT('Origin',(0.,0.,0.));
#16626=CARTESIAN_POINT('',(-0.523653836874034,0.,-0.315240018494132));
#16627=CARTESIAN_POINT('Origin',(-0.478711351753049,0.,-0.347804155687524));
#16628=CARTESIAN_POINT('',(-0.461629008549572,0.,-0.40060987082025));
#16629=CARTESIAN_POINT('Origin',(0.,0.,0.));
#16630=CARTESIAN_POINT('',(-0.40060987082025,0.,-0.461629008549572));
#16631=CARTESIAN_POINT('Origin',(-0.347804155687524,0.,-0.478711351753049));
#16632=CARTESIAN_POINT('',(-0.315240018494132,0.,-0.523653836874034));
#16633=CARTESIAN_POINT('Origin',(0.,0.,0.));
#16634=CARTESIAN_POINT('',(-0.238351419397483,0.,-0.562830534889751));
#16635=CARTESIAN_POINT('Origin',(-0.182851465569258,0.,-0.562758945330873));
#16636=CARTESIAN_POINT('',(-0.137993139022126,0.,-0.595438916863769));
#16637=CARTESIAN_POINT('Origin',(0.,0.,0.));
#16638=CARTESIAN_POINT('',(-0.0527614703521,0.,-0.608938287003997));
#16639=CARTESIAN_POINT('Origin',(3.6232386261108E-17,0.,-0.591719772367581));
#16640=CARTESIAN_POINT('',(0.0527614703521001,0.,-0.608938287003997));
#16641=CARTESIAN_POINT('Origin',(0.,0.,0.));
#16642=CARTESIAN_POINT('',(0.137993139022126,0.,-0.595438916863769));
#16643=CARTESIAN_POINT('Origin',(0.182851465569258,0.,-0.562758945330873));
#16644=CARTESIAN_POINT('',(0.238351419397483,0.,-0.562830534889751));
#16645=CARTESIAN_POINT('Origin',(0.,0.,0.));
#16646=CARTESIAN_POINT('',(0.315240018494132,0.,-0.523653836874034));
#16647=CARTESIAN_POINT('Origin',(0.347804155687524,0.,-0.478711351753049));
#16648=CARTESIAN_POINT('',(0.40060987082025,0.,-0.461629008549572));
#16649=CARTESIAN_POINT('Origin',(0.,0.,0.));
#16650=CARTESIAN_POINT('',(0.461629008549572,0.,-0.40060987082025));
#16651=CARTESIAN_POINT('Origin',(0.478711351753049,0.,-0.347804155687524));
#16652=CARTESIAN_POINT('',(0.523653836874034,0.,-0.315240018494132));
#16653=CARTESIAN_POINT('Origin',(0.,0.,0.));
#16654=CARTESIAN_POINT('',(0.562830534889751,0.,-0.238351419397483));
#16655=CARTESIAN_POINT('Origin',(0.562758945330873,0.,-0.182851465569258));
#16656=CARTESIAN_POINT('',(0.595438916863769,0.,-0.137993139022126));
#16657=CARTESIAN_POINT('Origin',(0.,0.,0.));
#16658=CARTESIAN_POINT('',(0.608938287003997,0.,0.0527614703521001));
#16659=CARTESIAN_POINT('Origin',(0.591719772367581,0.,0.));
#16660=CARTESIAN_POINT('',(0.608938287003997,0.,-0.0527614703521001));
#16661=CARTESIAN_POINT('Origin',(0.,0.,0.));
#17770=UNCERTAINTY_MEASURE_WITH_UNIT(LENGTH_MEASURE(0.001),#17831,
'DISTANCE_ACCURACY_VALUE',
'Maximum model space distance between geometric entities at asserted c
onnectivities');
#17780=UNCERTAINTY_MEASURE_WITH_UNIT(LENGTH_MEASURE(0.001),#17831,
'DISTANCE_ACCURACY_VALUE',
'Maximum model space distance between geometric entities at asserted c
onnectivities');
#17820=(
GEOMETRIC_REPRESENTATION_CONTEXT(3)
GLOBAL_UNCERTAINTY_ASSIGNED_CONTEXT((#17770))
GLOBAL_UNIT_ASSIGNED_CONTEXT((#17831,#17833,#17834))
REPRESENTATION_CONTEXT('','3D')
);
#17830=(
GEOMETRIC_REPRESENTATION_CONTEXT(3)
GLOBAL_UNCERTAINTY_ASSIGNED_CONTEXT((#17780))
GLOBAL_UNIT_ASSIGNED_CONTEXT((#17831,#17833,#17834))
REPRESENTATION_CONTEXT('','3D')
);
#17831=(
LENGTH_UNIT()
NAMED_UNIT(*)
SI_UNIT(.CENTI.,.METRE.)
);
#17833=(
NAMED_UNIT(*)
PLANE_ANGLE_UNIT()
SI_UNIT($,.RADIAN.)
);
#17834=(
NAMED_UNIT(*)
SI_UNIT($,.STERADIAN.)
SOLID_ANGLE_UNIT()
);
#17874=SHAPE_DEFINITION_REPRESENTATION(#17933,#18045);
#17933=PRODUCT_DEFINITION_SHAPE('',$,#18095);
#18045=SHAPE_REPRESENTATION('',(#10258),#17820);
#18055=PRODUCT_DEFINITION_CONTEXT('part definition',#18204,'design');
#18095=PRODUCT_DEFINITION(
'Timing Pulley - 2 mm Pitch, 20 Teeth, 8 mm Bore',
'Timing Pulley - 2 mm Pitch, 20 Teeth, 8 mm Bore',#18144,#18055);
#18144=PRODUCT_DEFINITION_FORMATION('',$,#18245);
#18204=APPLICATION_CONTEXT(
'Core Data for Automotive Mechanical Design Process');
#18205=PRODUCT_CONTEXT('part definition',#18204,'mechanical');
#18245=PRODUCT('Timing Pulley - 2 mm Pitch, 20 Teeth, 8 mm Bore',
'Timing Pulley - 2 mm Pitch, 20 Teeth, 8 mm Bore',
'Timing Pulley - 2 mm Pitch, 20 Teeth, 8 mm Bore',(#18205));
#18325=COLOUR_RGB('Off White',0.89,0.88,0.83);
#18326=FILL_AREA_STYLE_COLOUR('',#18325);
#18327=FILL_AREA_STYLE('',(#18326));
#18328=SURFACE_STYLE_FILL_AREA(#18327);
#18329=SURFACE_SIDE_STYLE('',(#18328));
#18330=SURFACE_STYLE_USAGE(.BOTH.,#18329);
#18331=PRESENTATION_STYLE_ASSIGNMENT((#18330));
ENDSEC;
END-ISO-10303-21;
